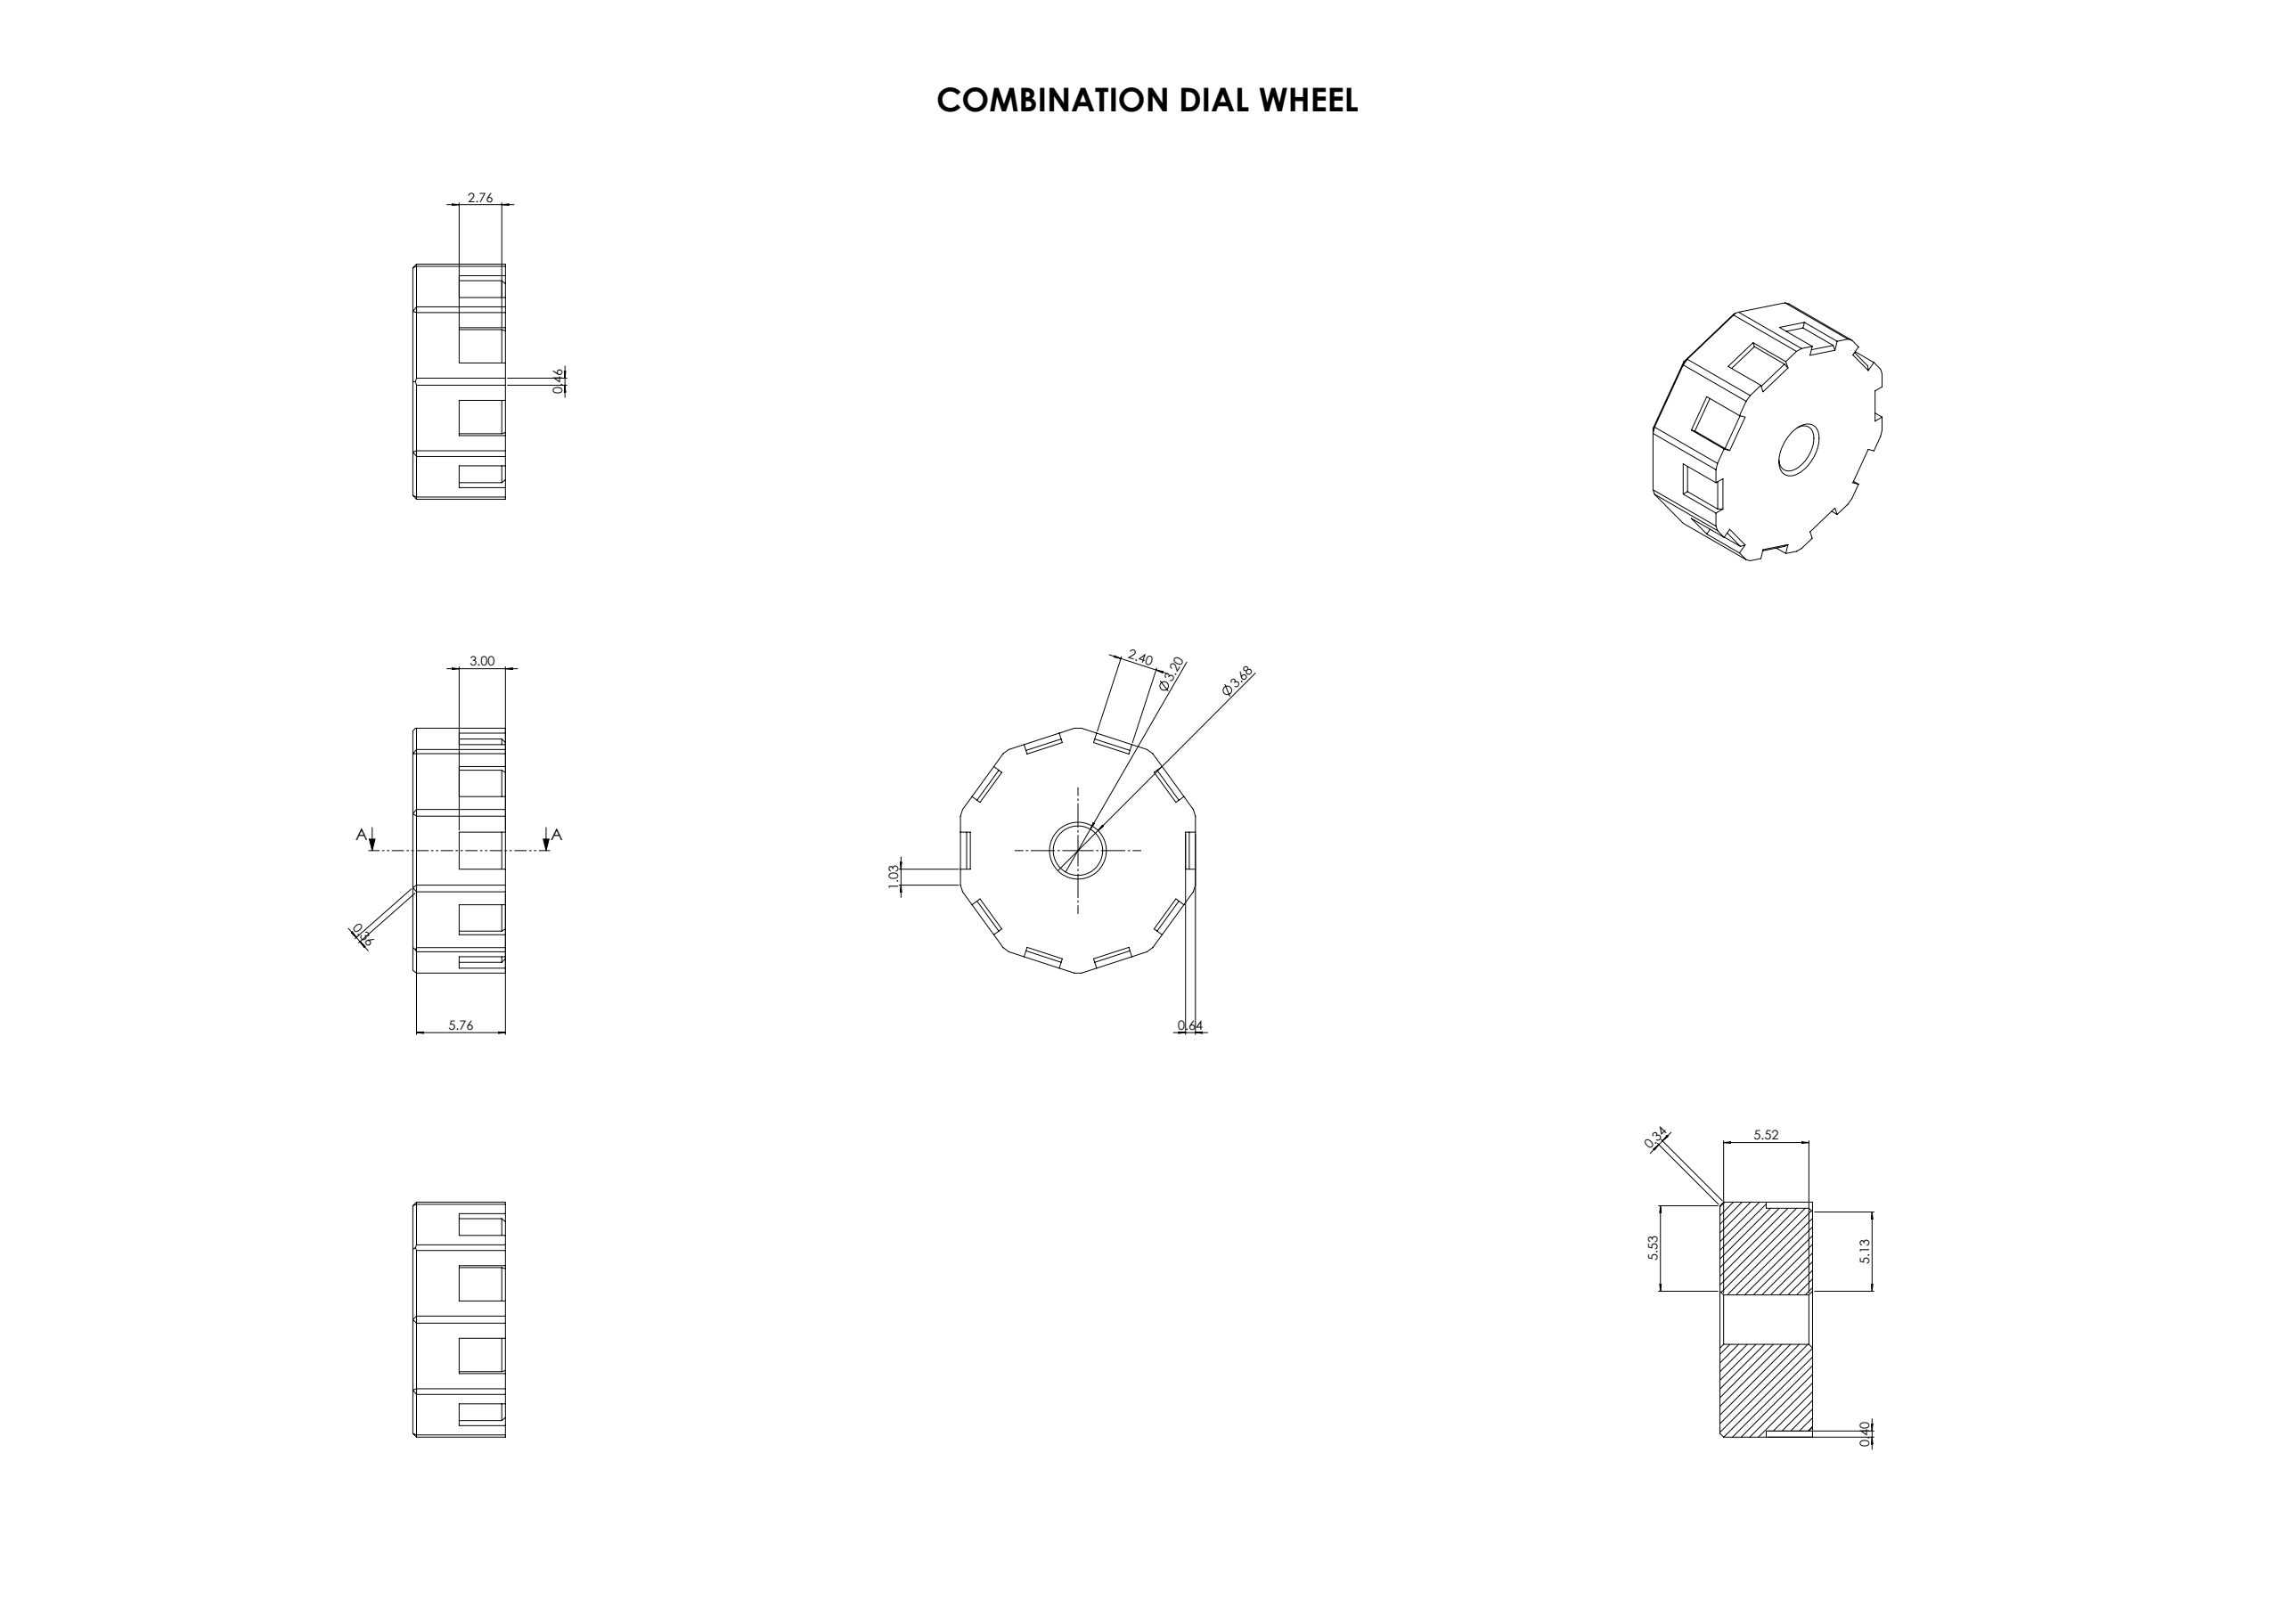
ISO-10303-21;
HEADER;
/* Generated by software containing ST-Developer
 * from STEP Tools, Inc. (www.steptools.com) 
 */

FILE_DESCRIPTION(
/* description */ (''),
/* implementation_level */ '2;1');

FILE_NAME(
/* name */ '10_Combination_Dial_Wheel.step',
/* time_stamp */ '2026-10-25T01:30:15-07:00',
/* author */ (''),
/* organization */ (''),
/* preprocessor_version */ 'ST-DEVELOPER v20.2',
/* originating_system */ 'Autodesk Translation Framework v15.15.0.0',
/* authorisation */ '');

FILE_SCHEMA (('AUTOMOTIVE_DESIGN { 1 0 10303 214 3 1 1 }'));
ENDSEC;

DATA;
#10=MECHANICAL_DESIGN_GEOMETRIC_PRESENTATION_REPRESENTATION('',(#576),#32309);
#548=SHAPE_REPRESENTATION_RELATIONSHIP('SRR','None',#32375,#562);
#562=ADVANCED_BREP_SHAPE_REPRESENTATION('',(#590),#32308);
#576=STYLED_ITEM('',(#32488),#590);
#590=MANIFOLD_SOLID_BREP('Body1',#13817);
#645=FACE_BOUND('',#2804,.T.);
#646=FACE_BOUND('',#2807,.T.);
#772=CYLINDRICAL_SURFACE('',#14893,1.6);
#1093=CIRCLE('',#14891,1.6);
#1094=CIRCLE('',#14892,1.84);
#1095=CIRCLE('',#14894,1.6);
#1096=CIRCLE('',#14897,1.84);
#1240=CONICAL_SURFACE('',#14890,1.72,0.785398163397448);
#1241=CONICAL_SURFACE('',#14896,1.72,0.785398163397448);
#1948=FACE_OUTER_BOUND('',#2801,.T.);
#1949=FACE_OUTER_BOUND('',#2802,.T.);
#1950=FACE_OUTER_BOUND('',#2803,.T.);
#1951=FACE_OUTER_BOUND('',#2805,.T.);
#1952=FACE_OUTER_BOUND('',#2806,.T.);
#1953=FACE_OUTER_BOUND('',#2808,.T.);
#1954=FACE_OUTER_BOUND('',#2809,.T.);
#1955=FACE_OUTER_BOUND('',#2810,.T.);
#1956=FACE_OUTER_BOUND('',#2811,.T.);
#1957=FACE_OUTER_BOUND('',#2812,.T.);
#1958=FACE_OUTER_BOUND('',#2813,.T.);
#1959=FACE_OUTER_BOUND('',#2814,.T.);
#1960=FACE_OUTER_BOUND('',#2815,.T.);
#1961=FACE_OUTER_BOUND('',#2816,.T.);
#1962=FACE_OUTER_BOUND('',#2817,.T.);
#1963=FACE_OUTER_BOUND('',#2818,.T.);
#1964=FACE_OUTER_BOUND('',#2819,.T.);
#1965=FACE_OUTER_BOUND('',#2820,.T.);
#1966=FACE_OUTER_BOUND('',#2821,.T.);
#1967=FACE_OUTER_BOUND('',#2822,.T.);
#1968=FACE_OUTER_BOUND('',#2823,.T.);
#1969=FACE_OUTER_BOUND('',#2824,.T.);
#1970=FACE_OUTER_BOUND('',#2825,.T.);
#1971=FACE_OUTER_BOUND('',#2826,.T.);
#1972=FACE_OUTER_BOUND('',#2827,.T.);
#1973=FACE_OUTER_BOUND('',#2828,.T.);
#1974=FACE_OUTER_BOUND('',#2829,.T.);
#1975=FACE_OUTER_BOUND('',#2830,.T.);
#1976=FACE_OUTER_BOUND('',#2831,.T.);
#1977=FACE_OUTER_BOUND('',#2832,.T.);
#1978=FACE_OUTER_BOUND('',#2833,.T.);
#1979=FACE_OUTER_BOUND('',#2834,.T.);
#1980=FACE_OUTER_BOUND('',#2835,.T.);
#1981=FACE_OUTER_BOUND('',#2836,.T.);
#1982=FACE_OUTER_BOUND('',#2837,.T.);
#1983=FACE_OUTER_BOUND('',#2838,.T.);
#1984=FACE_OUTER_BOUND('',#2839,.T.);
#1985=FACE_OUTER_BOUND('',#2840,.T.);
#1986=FACE_OUTER_BOUND('',#2841,.T.);
#1987=FACE_OUTER_BOUND('',#2842,.T.);
#1988=FACE_OUTER_BOUND('',#2843,.T.);
#1989=FACE_OUTER_BOUND('',#2844,.T.);
#1990=FACE_OUTER_BOUND('',#2845,.T.);
#1991=FACE_OUTER_BOUND('',#2846,.T.);
#1992=FACE_OUTER_BOUND('',#2847,.T.);
#1993=FACE_OUTER_BOUND('',#2848,.T.);
#1994=FACE_OUTER_BOUND('',#2849,.T.);
#1995=FACE_OUTER_BOUND('',#2850,.T.);
#1996=FACE_OUTER_BOUND('',#2851,.T.);
#1997=FACE_OUTER_BOUND('',#2852,.T.);
#1998=FACE_OUTER_BOUND('',#2853,.T.);
#1999=FACE_OUTER_BOUND('',#2854,.T.);
#2000=FACE_OUTER_BOUND('',#2855,.T.);
#2001=FACE_OUTER_BOUND('',#2856,.T.);
#2002=FACE_OUTER_BOUND('',#2857,.T.);
#2003=FACE_OUTER_BOUND('',#2858,.T.);
#2004=FACE_OUTER_BOUND('',#2859,.T.);
#2005=FACE_OUTER_BOUND('',#2860,.T.);
#2006=FACE_OUTER_BOUND('',#2861,.T.);
#2007=FACE_OUTER_BOUND('',#2862,.T.);
#2008=FACE_OUTER_BOUND('',#2863,.T.);
#2009=FACE_OUTER_BOUND('',#2864,.T.);
#2010=FACE_OUTER_BOUND('',#2865,.T.);
#2011=FACE_OUTER_BOUND('',#2866,.T.);
#2012=FACE_OUTER_BOUND('',#2867,.T.);
#2013=FACE_OUTER_BOUND('',#2868,.T.);
#2014=FACE_OUTER_BOUND('',#2869,.T.);
#2015=FACE_OUTER_BOUND('',#2870,.T.);
#2016=FACE_OUTER_BOUND('',#2871,.T.);
#2017=FACE_OUTER_BOUND('',#2872,.T.);
#2018=FACE_OUTER_BOUND('',#2873,.T.);
#2019=FACE_OUTER_BOUND('',#2874,.T.);
#2020=FACE_OUTER_BOUND('',#2875,.T.);
#2021=FACE_OUTER_BOUND('',#2876,.T.);
#2022=FACE_OUTER_BOUND('',#2877,.T.);
#2023=FACE_OUTER_BOUND('',#2878,.T.);
#2024=FACE_OUTER_BOUND('',#2879,.T.);
#2025=FACE_OUTER_BOUND('',#2880,.T.);
#2026=FACE_OUTER_BOUND('',#2881,.T.);
#2027=FACE_OUTER_BOUND('',#2882,.T.);
#2028=FACE_OUTER_BOUND('',#2883,.T.);
#2029=FACE_OUTER_BOUND('',#2884,.T.);
#2030=FACE_OUTER_BOUND('',#2885,.T.);
#2031=FACE_OUTER_BOUND('',#2886,.T.);
#2032=FACE_OUTER_BOUND('',#2887,.T.);
#2033=FACE_OUTER_BOUND('',#2888,.T.);
#2034=FACE_OUTER_BOUND('',#2889,.T.);
#2035=FACE_OUTER_BOUND('',#2890,.T.);
#2036=FACE_OUTER_BOUND('',#2891,.T.);
#2037=FACE_OUTER_BOUND('',#2892,.T.);
#2038=FACE_OUTER_BOUND('',#2893,.T.);
#2039=FACE_OUTER_BOUND('',#2894,.T.);
#2040=FACE_OUTER_BOUND('',#2895,.T.);
#2801=EDGE_LOOP('',(#12111,#12112,#12113,#12114));
#2802=EDGE_LOOP('',(#12115,#12116,#12117,#12118));
#2803=EDGE_LOOP('',(#12119,#12120,#12121,#12122,#12123,#12124,#12125,#12126,
#12127,#12128));
#2804=EDGE_LOOP('',(#12129));
#2805=EDGE_LOOP('',(#12130,#12131,#12132,#12133));
#2806=EDGE_LOOP('',(#12134,#12135,#12136,#12137,#12138,#12139,#12140,#12141,
#12142,#12143,#12144,#12145,#12146,#12147,#12148,#12149,#12150,#12151,#12152,
#12153,#12154,#12155,#12156,#12157,#12158,#12159,#12160,#12161,#12162,#12163,
#12164,#12165,#12166,#12167,#12168,#12169,#12170,#12171,#12172,#12173,#12174,
#12175,#12176,#12177,#12178,#12179,#12180,#12181,#12182,#12183,#12184,#12185,
#12186,#12187,#12188,#12189,#12190,#12191,#12192,#12193));
#2807=EDGE_LOOP('',(#12194));
#2808=EDGE_LOOP('',(#12195,#12196,#12197,#12198));
#2809=EDGE_LOOP('',(#12199,#12200,#12201,#12202));
#2810=EDGE_LOOP('',(#12203,#12204,#12205,#12206));
#2811=EDGE_LOOP('',(#12207,#12208,#12209,#12210));
#2812=EDGE_LOOP('',(#12211,#12212,#12213,#12214));
#2813=EDGE_LOOP('',(#12215,#12216,#12217,#12218));
#2814=EDGE_LOOP('',(#12219,#12220,#12221));
#2815=EDGE_LOOP('',(#12222,#12223,#12224,#12225,#12226));
#2816=EDGE_LOOP('',(#12227,#12228,#12229));
#2817=EDGE_LOOP('',(#12230,#12231,#12232,#12233));
#2818=EDGE_LOOP('',(#12234,#12235,#12236));
#2819=EDGE_LOOP('',(#12237,#12238,#12239,#12240));
#2820=EDGE_LOOP('',(#12241,#12242,#12243,#12244,#12245));
#2821=EDGE_LOOP('',(#12246,#12247,#12248,#12249));
#2822=EDGE_LOOP('',(#12250,#12251,#12252,#12253));
#2823=EDGE_LOOP('',(#12254,#12255,#12256,#12257));
#2824=EDGE_LOOP('',(#12258,#12259,#12260,#12261,#12262,#12263,#12264,#12265));
#2825=EDGE_LOOP('',(#12266,#12267,#12268,#12269,#12270,#12271,#12272,#12273));
#2826=EDGE_LOOP('',(#12274,#12275,#12276,#12277,#12278,#12279,#12280,#12281));
#2827=EDGE_LOOP('',(#12282,#12283,#12284,#12285,#12286));
#2828=EDGE_LOOP('',(#12287,#12288,#12289,#12290,#12291));
#2829=EDGE_LOOP('',(#12292,#12293,#12294,#12295));
#2830=EDGE_LOOP('',(#12296,#12297,#12298,#12299));
#2831=EDGE_LOOP('',(#12300,#12301,#12302,#12303));
#2832=EDGE_LOOP('',(#12304,#12305,#12306,#12307));
#2833=EDGE_LOOP('',(#12308,#12309,#12310,#12311));
#2834=EDGE_LOOP('',(#12312,#12313,#12314,#12315));
#2835=EDGE_LOOP('',(#12316,#12317,#12318,#12319));
#2836=EDGE_LOOP('',(#12320,#12321,#12322,#12323));
#2837=EDGE_LOOP('',(#12324,#12325,#12326,#12327));
#2838=EDGE_LOOP('',(#12328,#12329,#12330,#12331));
#2839=EDGE_LOOP('',(#12332,#12333,#12334,#12335));
#2840=EDGE_LOOP('',(#12336,#12337,#12338,#12339));
#2841=EDGE_LOOP('',(#12340,#12341,#12342));
#2842=EDGE_LOOP('',(#12343,#12344,#12345));
#2843=EDGE_LOOP('',(#12346,#12347,#12348,#12349));
#2844=EDGE_LOOP('',(#12350,#12351,#12352));
#2845=EDGE_LOOP('',(#12353,#12354,#12355,#12356));
#2846=EDGE_LOOP('',(#12357,#12358,#12359));
#2847=EDGE_LOOP('',(#12360,#12361,#12362,#12363));
#2848=EDGE_LOOP('',(#12364,#12365,#12366));
#2849=EDGE_LOOP('',(#12367,#12368,#12369,#12370,#12371));
#2850=EDGE_LOOP('',(#12372,#12373,#12374,#12375));
#2851=EDGE_LOOP('',(#12376,#12377,#12378,#12379));
#2852=EDGE_LOOP('',(#12380,#12381,#12382,#12383,#12384));
#2853=EDGE_LOOP('',(#12385,#12386,#12387,#12388));
#2854=EDGE_LOOP('',(#12389,#12390,#12391,#12392));
#2855=EDGE_LOOP('',(#12393,#12394,#12395,#12396));
#2856=EDGE_LOOP('',(#12397,#12398,#12399,#12400));
#2857=EDGE_LOOP('',(#12401,#12402,#12403,#12404,#12405,#12406,#12407,#12408));
#2858=EDGE_LOOP('',(#12409,#12410,#12411,#12412,#12413,#12414,#12415,#12416));
#2859=EDGE_LOOP('',(#12417,#12418,#12419,#12420,#12421,#12422,#12423,#12424));
#2860=EDGE_LOOP('',(#12425,#12426,#12427,#12428,#12429,#12430,#12431,#12432));
#2861=EDGE_LOOP('',(#12433,#12434,#12435,#12436,#12437,#12438,#12439,#12440));
#2862=EDGE_LOOP('',(#12441,#12442,#12443,#12444));
#2863=EDGE_LOOP('',(#12445,#12446,#12447,#12448));
#2864=EDGE_LOOP('',(#12449,#12450,#12451,#12452));
#2865=EDGE_LOOP('',(#12453,#12454,#12455,#12456,#12457));
#2866=EDGE_LOOP('',(#12458,#12459,#12460,#12461,#12462));
#2867=EDGE_LOOP('',(#12463,#12464,#12465,#12466,#12467,#12468,#12469,#12470));
#2868=EDGE_LOOP('',(#12471,#12472,#12473,#12474));
#2869=EDGE_LOOP('',(#12475,#12476,#12477,#12478,#12479));
#2870=EDGE_LOOP('',(#12480,#12481,#12482,#12483,#12484));
#2871=EDGE_LOOP('',(#12485,#12486,#12487,#12488));
#2872=EDGE_LOOP('',(#12489,#12490,#12491,#12492,#12493));
#2873=EDGE_LOOP('',(#12494,#12495,#12496,#12497,#12498));
#2874=EDGE_LOOP('',(#12499,#12500,#12501,#12502));
#2875=EDGE_LOOP('',(#12503,#12504,#12505,#12506,#12507));
#2876=EDGE_LOOP('',(#12508,#12509,#12510,#12511,#12512));
#2877=EDGE_LOOP('',(#12513,#12514,#12515,#12516));
#2878=EDGE_LOOP('',(#12517,#12518,#12519,#12520,#12521));
#2879=EDGE_LOOP('',(#12522,#12523,#12524,#12525,#12526));
#2880=EDGE_LOOP('',(#12527,#12528,#12529,#12530));
#2881=EDGE_LOOP('',(#12531,#12532,#12533,#12534,#12535));
#2882=EDGE_LOOP('',(#12536,#12537,#12538,#12539,#12540));
#2883=EDGE_LOOP('',(#12541,#12542,#12543,#12544));
#2884=EDGE_LOOP('',(#12545,#12546,#12547,#12548,#12549));
#2885=EDGE_LOOP('',(#12550,#12551,#12552,#12553,#12554));
#2886=EDGE_LOOP('',(#12555,#12556,#12557,#12558));
#2887=EDGE_LOOP('',(#12559,#12560,#12561,#12562,#12563));
#2888=EDGE_LOOP('',(#12564,#12565,#12566,#12567,#12568));
#2889=EDGE_LOOP('',(#12569,#12570,#12571,#12572));
#2890=EDGE_LOOP('',(#12573,#12574,#12575,#12576,#12577));
#2891=EDGE_LOOP('',(#12578,#12579,#12580,#12581,#12582));
#2892=EDGE_LOOP('',(#12583,#12584,#12585,#12586,#12587));
#2893=EDGE_LOOP('',(#12588,#12589,#12590,#12591,#12592));
#2894=EDGE_LOOP('',(#12593,#12594,#12595,#12596));
#2895=EDGE_LOOP('',(#12597,#12598,#12599,#12600,#12601,#12602,#12603,#12604));
#3964=LINE('',#31769,#5275);
#3965=LINE('',#31774,#5276);
#3966=LINE('',#31778,#5277);
#3967=LINE('',#31780,#5278);
#3968=LINE('',#31782,#5279);
#3969=LINE('',#31784,#5280);
#3970=LINE('',#31786,#5281);
#3971=LINE('',#31788,#5282);
#3972=LINE('',#31790,#5283);
#3973=LINE('',#31792,#5284);
#3974=LINE('',#31794,#5285);
#3975=LINE('',#31795,#5286);
#3976=LINE('',#31799,#5287);
#3977=LINE('',#31803,#5288);
#3978=LINE('',#31805,#5289);
#3979=LINE('',#31807,#5290);
#3980=LINE('',#31809,#5291);
#3981=LINE('',#31811,#5292);
#3982=LINE('',#31813,#5293);
#3983=LINE('',#31815,#5294);
#3984=LINE('',#31817,#5295);
#3985=LINE('',#31819,#5296);
#3986=LINE('',#31821,#5297);
#3987=LINE('',#31823,#5298);
#3988=LINE('',#31825,#5299);
#3989=LINE('',#31827,#5300);
#3990=LINE('',#31829,#5301);
#3991=LINE('',#31831,#5302);
#3992=LINE('',#31833,#5303);
#3993=LINE('',#31835,#5304);
#3994=LINE('',#31837,#5305);
#3995=LINE('',#31839,#5306);
#3996=LINE('',#31841,#5307);
#3997=LINE('',#31843,#5308);
#3998=LINE('',#31845,#5309);
#3999=LINE('',#31847,#5310);
#4000=LINE('',#31849,#5311);
#4001=LINE('',#31851,#5312);
#4002=LINE('',#31853,#5313);
#4003=LINE('',#31855,#5314);
#4004=LINE('',#31857,#5315);
#4005=LINE('',#31859,#5316);
#4006=LINE('',#31861,#5317);
#4007=LINE('',#31863,#5318);
#4008=LINE('',#31865,#5319);
#4009=LINE('',#31867,#5320);
#4010=LINE('',#31869,#5321);
#4011=LINE('',#31871,#5322);
#4012=LINE('',#31873,#5323);
#4013=LINE('',#31875,#5324);
#4014=LINE('',#31877,#5325);
#4015=LINE('',#31879,#5326);
#4016=LINE('',#31881,#5327);
#4017=LINE('',#31883,#5328);
#4018=LINE('',#31885,#5329);
#4019=LINE('',#31887,#5330);
#4020=LINE('',#31889,#5331);
#4021=LINE('',#31891,#5332);
#4022=LINE('',#31893,#5333);
#4023=LINE('',#31895,#5334);
#4024=LINE('',#31897,#5335);
#4025=LINE('',#31899,#5336);
#4026=LINE('',#31901,#5337);
#4027=LINE('',#31903,#5338);
#4028=LINE('',#31905,#5339);
#4029=LINE('',#31907,#5340);
#4030=LINE('',#31909,#5341);
#4031=LINE('',#31911,#5342);
#4032=LINE('',#31913,#5343);
#4033=LINE('',#31915,#5344);
#4034=LINE('',#31917,#5345);
#4035=LINE('',#31919,#5346);
#4036=LINE('',#31920,#5347);
#4037=LINE('',#31923,#5348);
#4038=LINE('',#31925,#5349);
#4039=LINE('',#31926,#5350);
#4040=LINE('',#31929,#5351);
#4041=LINE('',#31931,#5352);
#4042=LINE('',#31932,#5353);
#4043=LINE('',#31935,#5354);
#4044=LINE('',#31937,#5355);
#4045=LINE('',#31938,#5356);
#4046=LINE('',#31941,#5357);
#4047=LINE('',#31943,#5358);
#4048=LINE('',#31944,#5359);
#4049=LINE('',#31947,#5360);
#4050=LINE('',#31949,#5361);
#4051=LINE('',#31950,#5362);
#4052=LINE('',#31953,#5363);
#4053=LINE('',#31955,#5364);
#4054=LINE('',#31956,#5365);
#4055=LINE('',#31960,#5366);
#4056=LINE('',#31961,#5367);
#4057=LINE('',#31962,#5368);
#4058=LINE('',#31965,#5369);
#4059=LINE('',#31967,#5370);
#4060=LINE('',#31968,#5371);
#4061=LINE('',#31972,#5372);
#4062=LINE('',#31973,#5373);
#4063=LINE('',#31974,#5374);
#4064=LINE('',#31976,#5375);
#4065=LINE('',#31980,#5376);
#4066=LINE('',#31981,#5377);
#4067=LINE('',#31982,#5378);
#4068=LINE('',#31984,#5379);
#4069=LINE('',#31988,#5380);
#4070=LINE('',#31989,#5381);
#4071=LINE('',#31990,#5382);
#4072=LINE('',#31992,#5383);
#4073=LINE('',#31993,#5384);
#4074=LINE('',#31995,#5385);
#4075=LINE('',#31996,#5386);
#4076=LINE('',#31998,#5387);
#4077=LINE('',#31999,#5388);
#4078=LINE('',#32002,#5389);
#4079=LINE('',#32004,#5390);
#4080=LINE('',#32005,#5391);
#4081=LINE('',#32008,#5392);
#4082=LINE('',#32010,#5393);
#4083=LINE('',#32011,#5394);
#4084=LINE('',#32013,#5395);
#4085=LINE('',#32015,#5396);
#4086=LINE('',#32017,#5397);
#4087=LINE('',#32018,#5398);
#4088=LINE('',#32021,#5399);
#4089=LINE('',#32022,#5400);
#4090=LINE('',#32025,#5401);
#4091=LINE('',#32026,#5402);
#4092=LINE('',#32029,#5403);
#4093=LINE('',#32031,#5404);
#4094=LINE('',#32032,#5405);
#4095=LINE('',#32035,#5406);
#4096=LINE('',#32037,#5407);
#4097=LINE('',#32038,#5408);
#4098=LINE('',#32041,#5409);
#4099=LINE('',#32043,#5410);
#4100=LINE('',#32044,#5411);
#4101=LINE('',#32047,#5412);
#4102=LINE('',#32049,#5413);
#4103=LINE('',#32050,#5414);
#4104=LINE('',#32053,#5415);
#4105=LINE('',#32055,#5416);
#4106=LINE('',#32056,#5417);
#4107=LINE('',#32059,#5418);
#4108=LINE('',#32061,#5419);
#4109=LINE('',#32062,#5420);
#4110=LINE('',#32065,#5421);
#4111=LINE('',#32067,#5422);
#4112=LINE('',#32068,#5423);
#4113=LINE('',#32071,#5424);
#4114=LINE('',#32073,#5425);
#4115=LINE('',#32074,#5426);
#4116=LINE('',#32077,#5427);
#4117=LINE('',#32079,#5428);
#4118=LINE('',#32080,#5429);
#4119=LINE('',#32083,#5430);
#4120=LINE('',#32085,#5431);
#4121=LINE('',#32086,#5432);
#4122=LINE('',#32089,#5433);
#4123=LINE('',#32091,#5434);
#4124=LINE('',#32092,#5435);
#4125=LINE('',#32095,#5436);
#4126=LINE('',#32097,#5437);
#4127=LINE('',#32098,#5438);
#4128=LINE('',#32101,#5439);
#4129=LINE('',#32102,#5440);
#4130=LINE('',#32106,#5441);
#4131=LINE('',#32107,#5442);
#4132=LINE('',#32108,#5443);
#4133=LINE('',#32110,#5444);
#4134=LINE('',#32114,#5445);
#4135=LINE('',#32115,#5446);
#4136=LINE('',#32116,#5447);
#4137=LINE('',#32118,#5448);
#4138=LINE('',#32122,#5449);
#4139=LINE('',#32123,#5450);
#4140=LINE('',#32124,#5451);
#4141=LINE('',#32126,#5452);
#4142=LINE('',#32129,#5453);
#4143=LINE('',#32131,#5454);
#4144=LINE('',#32132,#5455);
#4145=LINE('',#32135,#5456);
#4146=LINE('',#32136,#5457);
#4147=LINE('',#32138,#5458);
#4148=LINE('',#32139,#5459);
#4149=LINE('',#32141,#5460);
#4150=LINE('',#32143,#5461);
#4151=LINE('',#32144,#5462);
#4152=LINE('',#32146,#5463);
#4153=LINE('',#32147,#5464);
#4154=LINE('',#32149,#5465);
#4155=LINE('',#32150,#5466);
#4156=LINE('',#32152,#5467);
#4157=LINE('',#32153,#5468);
#4158=LINE('',#32155,#5469);
#4159=LINE('',#32156,#5470);
#4160=LINE('',#32159,#5471);
#4161=LINE('',#32161,#5472);
#4162=LINE('',#32162,#5473);
#4163=LINE('',#32165,#5474);
#4164=LINE('',#32167,#5475);
#4165=LINE('',#32168,#5476);
#4166=LINE('',#32171,#5477);
#4167=LINE('',#32173,#5478);
#4168=LINE('',#32174,#5479);
#4169=LINE('',#32177,#5480);
#4170=LINE('',#32179,#5481);
#4171=LINE('',#32180,#5482);
#4172=LINE('',#32183,#5483);
#4173=LINE('',#32185,#5484);
#4174=LINE('',#32186,#5485);
#4175=LINE('',#32189,#5486);
#4176=LINE('',#32191,#5487);
#4177=LINE('',#32192,#5488);
#4178=LINE('',#32195,#5489);
#4179=LINE('',#32197,#5490);
#4180=LINE('',#32198,#5491);
#4181=LINE('',#32202,#5492);
#4182=LINE('',#32203,#5493);
#4183=LINE('',#32204,#5494);
#4184=LINE('',#32206,#5495);
#4185=LINE('',#32208,#5496);
#4186=LINE('',#32211,#5497);
#4187=LINE('',#32212,#5498);
#4188=LINE('',#32216,#5499);
#4189=LINE('',#32217,#5500);
#4190=LINE('',#32221,#5501);
#4191=LINE('',#32222,#5502);
#4192=LINE('',#32226,#5503);
#4193=LINE('',#32227,#5504);
#4194=LINE('',#32231,#5505);
#4195=LINE('',#32232,#5506);
#4196=LINE('',#32236,#5507);
#4197=LINE('',#32237,#5508);
#4198=LINE('',#32241,#5509);
#4199=LINE('',#32242,#5510);
#4200=LINE('',#32246,#5511);
#4201=LINE('',#32247,#5512);
#4202=LINE('',#32252,#5513);
#4203=LINE('',#32253,#5514);
#4204=LINE('',#32256,#5515);
#4205=LINE('',#32257,#5516);
#4206=LINE('',#32259,#5517);
#5275=VECTOR('',#17910,1.72);
#5276=VECTOR('',#17917,1.6);
#5277=VECTOR('',#17920,10.);
#5278=VECTOR('',#17921,10.);
#5279=VECTOR('',#17922,10.);
#5280=VECTOR('',#17923,10.);
#5281=VECTOR('',#17924,10.);
#5282=VECTOR('',#17925,10.);
#5283=VECTOR('',#17926,10.);
#5284=VECTOR('',#17927,10.);
#5285=VECTOR('',#17928,10.);
#5286=VECTOR('',#17929,10.);
#5287=VECTOR('',#17934,1.72);
#5288=VECTOR('',#17937,10.);
#5289=VECTOR('',#17938,10.);
#5290=VECTOR('',#17939,10.);
#5291=VECTOR('',#17940,10.);
#5292=VECTOR('',#17941,10.);
#5293=VECTOR('',#17942,10.);
#5294=VECTOR('',#17943,10.);
#5295=VECTOR('',#17944,10.);
#5296=VECTOR('',#17945,10.);
#5297=VECTOR('',#17946,10.);
#5298=VECTOR('',#17947,10.);
#5299=VECTOR('',#17948,10.);
#5300=VECTOR('',#17949,10.);
#5301=VECTOR('',#17950,10.);
#5302=VECTOR('',#17951,10.);
#5303=VECTOR('',#17952,10.);
#5304=VECTOR('',#17953,10.);
#5305=VECTOR('',#17954,10.);
#5306=VECTOR('',#17955,10.);
#5307=VECTOR('',#17956,10.);
#5308=VECTOR('',#17957,10.);
#5309=VECTOR('',#17958,10.);
#5310=VECTOR('',#17959,10.);
#5311=VECTOR('',#17960,10.);
#5312=VECTOR('',#17961,10.);
#5313=VECTOR('',#17962,10.);
#5314=VECTOR('',#17963,10.);
#5315=VECTOR('',#17964,10.);
#5316=VECTOR('',#17965,10.);
#5317=VECTOR('',#17966,10.);
#5318=VECTOR('',#17967,10.);
#5319=VECTOR('',#17968,10.);
#5320=VECTOR('',#17969,10.);
#5321=VECTOR('',#17970,10.);
#5322=VECTOR('',#17971,10.);
#5323=VECTOR('',#17972,10.);
#5324=VECTOR('',#17973,10.);
#5325=VECTOR('',#17974,10.);
#5326=VECTOR('',#17975,10.);
#5327=VECTOR('',#17976,10.);
#5328=VECTOR('',#17977,10.);
#5329=VECTOR('',#17978,10.);
#5330=VECTOR('',#17979,10.);
#5331=VECTOR('',#17980,10.);
#5332=VECTOR('',#17981,10.);
#5333=VECTOR('',#17982,10.);
#5334=VECTOR('',#17983,10.);
#5335=VECTOR('',#17984,10.);
#5336=VECTOR('',#17985,10.);
#5337=VECTOR('',#17986,10.);
#5338=VECTOR('',#17987,10.);
#5339=VECTOR('',#17988,10.);
#5340=VECTOR('',#17989,10.);
#5341=VECTOR('',#17990,10.);
#5342=VECTOR('',#17991,10.);
#5343=VECTOR('',#17992,10.);
#5344=VECTOR('',#17993,10.);
#5345=VECTOR('',#17994,10.);
#5346=VECTOR('',#17995,10.);
#5347=VECTOR('',#17996,10.);
#5348=VECTOR('',#17999,10.);
#5349=VECTOR('',#18000,10.);
#5350=VECTOR('',#18001,10.);
#5351=VECTOR('',#18004,10.);
#5352=VECTOR('',#18005,10.);
#5353=VECTOR('',#18006,10.);
#5354=VECTOR('',#18009,10.);
#5355=VECTOR('',#18010,10.);
#5356=VECTOR('',#18011,10.);
#5357=VECTOR('',#18014,10.);
#5358=VECTOR('',#18015,10.);
#5359=VECTOR('',#18016,10.);
#5360=VECTOR('',#18019,10.);
#5361=VECTOR('',#18020,10.);
#5362=VECTOR('',#18021,10.);
#5363=VECTOR('',#18024,10.);
#5364=VECTOR('',#18025,10.);
#5365=VECTOR('',#18026,10.);
#5366=VECTOR('',#18029,10.);
#5367=VECTOR('',#18030,10.);
#5368=VECTOR('',#18031,10.);
#5369=VECTOR('',#18034,10.);
#5370=VECTOR('',#18035,10.);
#5371=VECTOR('',#18036,10.);
#5372=VECTOR('',#18039,10.);
#5373=VECTOR('',#18040,10.);
#5374=VECTOR('',#18041,10.);
#5375=VECTOR('',#18044,10.);
#5376=VECTOR('',#18047,10.);
#5377=VECTOR('',#18048,10.);
#5378=VECTOR('',#18049,10.);
#5379=VECTOR('',#18052,10.);
#5380=VECTOR('',#18055,10.);
#5381=VECTOR('',#18056,10.);
#5382=VECTOR('',#18057,10.);
#5383=VECTOR('',#18060,10.);
#5384=VECTOR('',#18061,10.);
#5385=VECTOR('',#18064,10.);
#5386=VECTOR('',#18065,10.);
#5387=VECTOR('',#18068,10.);
#5388=VECTOR('',#18069,10.);
#5389=VECTOR('',#18072,10.);
#5390=VECTOR('',#18073,10.);
#5391=VECTOR('',#18074,10.);
#5392=VECTOR('',#18077,10.);
#5393=VECTOR('',#18078,10.);
#5394=VECTOR('',#18079,10.);
#5395=VECTOR('',#18082,10.);
#5396=VECTOR('',#18083,10.);
#5397=VECTOR('',#18084,10.);
#5398=VECTOR('',#18085,10.);
#5399=VECTOR('',#18088,10.);
#5400=VECTOR('',#18089,10.);
#5401=VECTOR('',#18092,10.);
#5402=VECTOR('',#18093,10.);
#5403=VECTOR('',#18096,10.);
#5404=VECTOR('',#18097,10.);
#5405=VECTOR('',#18098,10.);
#5406=VECTOR('',#18101,10.);
#5407=VECTOR('',#18102,10.);
#5408=VECTOR('',#18103,10.);
#5409=VECTOR('',#18106,10.);
#5410=VECTOR('',#18107,10.);
#5411=VECTOR('',#18108,10.);
#5412=VECTOR('',#18111,10.);
#5413=VECTOR('',#18112,10.);
#5414=VECTOR('',#18113,10.);
#5415=VECTOR('',#18116,10.);
#5416=VECTOR('',#18117,10.);
#5417=VECTOR('',#18118,10.);
#5418=VECTOR('',#18121,10.);
#5419=VECTOR('',#18122,10.);
#5420=VECTOR('',#18123,10.);
#5421=VECTOR('',#18126,10.);
#5422=VECTOR('',#18127,10.);
#5423=VECTOR('',#18128,10.);
#5424=VECTOR('',#18131,10.);
#5425=VECTOR('',#18132,10.);
#5426=VECTOR('',#18133,10.);
#5427=VECTOR('',#18136,10.);
#5428=VECTOR('',#18137,10.);
#5429=VECTOR('',#18138,10.);
#5430=VECTOR('',#18141,10.);
#5431=VECTOR('',#18142,10.);
#5432=VECTOR('',#18143,10.);
#5433=VECTOR('',#18146,10.);
#5434=VECTOR('',#18147,10.);
#5435=VECTOR('',#18148,10.);
#5436=VECTOR('',#18151,10.);
#5437=VECTOR('',#18152,10.);
#5438=VECTOR('',#18153,10.);
#5439=VECTOR('',#18156,10.);
#5440=VECTOR('',#18157,10.);
#5441=VECTOR('',#18160,10.);
#5442=VECTOR('',#18161,10.);
#5443=VECTOR('',#18162,10.);
#5444=VECTOR('',#18165,10.);
#5445=VECTOR('',#18168,10.);
#5446=VECTOR('',#18169,10.);
#5447=VECTOR('',#18170,10.);
#5448=VECTOR('',#18173,10.);
#5449=VECTOR('',#18176,10.);
#5450=VECTOR('',#18177,10.);
#5451=VECTOR('',#18178,10.);
#5452=VECTOR('',#18181,10.);
#5453=VECTOR('',#18184,10.);
#5454=VECTOR('',#18185,10.);
#5455=VECTOR('',#18186,10.);
#5456=VECTOR('',#18189,10.);
#5457=VECTOR('',#18190,10.);
#5458=VECTOR('',#18193,10.);
#5459=VECTOR('',#18194,10.);
#5460=VECTOR('',#18197,10.);
#5461=VECTOR('',#18200,10.);
#5462=VECTOR('',#18201,10.);
#5463=VECTOR('',#18204,10.);
#5464=VECTOR('',#18205,10.);
#5465=VECTOR('',#18208,10.);
#5466=VECTOR('',#18209,10.);
#5467=VECTOR('',#18212,10.);
#5468=VECTOR('',#18213,10.);
#5469=VECTOR('',#18216,10.);
#5470=VECTOR('',#18217,10.);
#5471=VECTOR('',#18220,10.);
#5472=VECTOR('',#18221,10.);
#5473=VECTOR('',#18222,10.);
#5474=VECTOR('',#18225,10.);
#5475=VECTOR('',#18226,10.);
#5476=VECTOR('',#18227,10.);
#5477=VECTOR('',#18230,10.);
#5478=VECTOR('',#18231,10.);
#5479=VECTOR('',#18232,10.);
#5480=VECTOR('',#18235,10.);
#5481=VECTOR('',#18236,10.);
#5482=VECTOR('',#18237,10.);
#5483=VECTOR('',#18240,10.);
#5484=VECTOR('',#18241,10.);
#5485=VECTOR('',#18242,10.);
#5486=VECTOR('',#18245,10.);
#5487=VECTOR('',#18246,10.);
#5488=VECTOR('',#18247,10.);
#5489=VECTOR('',#18250,10.);
#5490=VECTOR('',#18251,10.);
#5491=VECTOR('',#18252,10.);
#5492=VECTOR('',#18255,10.);
#5493=VECTOR('',#18256,10.);
#5494=VECTOR('',#18257,10.);
#5495=VECTOR('',#18260,10.);
#5496=VECTOR('',#18263,10.);
#5497=VECTOR('',#18268,10.);
#5498=VECTOR('',#18269,10.);
#5499=VECTOR('',#18276,10.);
#5500=VECTOR('',#18277,10.);
#5501=VECTOR('',#18284,10.);
#5502=VECTOR('',#18285,10.);
#5503=VECTOR('',#18292,10.);
#5504=VECTOR('',#18293,10.);
#5505=VECTOR('',#18300,10.);
#5506=VECTOR('',#18301,10.);
#5507=VECTOR('',#18308,10.);
#5508=VECTOR('',#18309,10.);
#5509=VECTOR('',#18316,10.);
#5510=VECTOR('',#18317,10.);
#5511=VECTOR('',#18324,10.);
#5512=VECTOR('',#18325,10.);
#5513=VECTOR('',#18332,10.);
#5514=VECTOR('',#18333,10.);
#5515=VECTOR('',#18336,10.);
#5516=VECTOR('',#18337,10.);
#5517=VECTOR('',#18340,10.);
#6560=VERTEX_POINT('',#31766);
#6561=VERTEX_POINT('',#31768);
#6562=VERTEX_POINT('',#31772);
#6563=VERTEX_POINT('',#31776);
#6564=VERTEX_POINT('',#31777);
#6565=VERTEX_POINT('',#31779);
#6566=VERTEX_POINT('',#31781);
#6567=VERTEX_POINT('',#31783);
#6568=VERTEX_POINT('',#31785);
#6569=VERTEX_POINT('',#31787);
#6570=VERTEX_POINT('',#31789);
#6571=VERTEX_POINT('',#31791);
#6572=VERTEX_POINT('',#31793);
#6573=VERTEX_POINT('',#31797);
#6574=VERTEX_POINT('',#31801);
#6575=VERTEX_POINT('',#31802);
#6576=VERTEX_POINT('',#31804);
#6577=VERTEX_POINT('',#31806);
#6578=VERTEX_POINT('',#31808);
#6579=VERTEX_POINT('',#31810);
#6580=VERTEX_POINT('',#31812);
#6581=VERTEX_POINT('',#31814);
#6582=VERTEX_POINT('',#31816);
#6583=VERTEX_POINT('',#31818);
#6584=VERTEX_POINT('',#31820);
#6585=VERTEX_POINT('',#31822);
#6586=VERTEX_POINT('',#31824);
#6587=VERTEX_POINT('',#31826);
#6588=VERTEX_POINT('',#31828);
#6589=VERTEX_POINT('',#31830);
#6590=VERTEX_POINT('',#31832);
#6591=VERTEX_POINT('',#31834);
#6592=VERTEX_POINT('',#31836);
#6593=VERTEX_POINT('',#31838);
#6594=VERTEX_POINT('',#31840);
#6595=VERTEX_POINT('',#31842);
#6596=VERTEX_POINT('',#31844);
#6597=VERTEX_POINT('',#31846);
#6598=VERTEX_POINT('',#31848);
#6599=VERTEX_POINT('',#31850);
#6600=VERTEX_POINT('',#31852);
#6601=VERTEX_POINT('',#31854);
#6602=VERTEX_POINT('',#31856);
#6603=VERTEX_POINT('',#31858);
#6604=VERTEX_POINT('',#31860);
#6605=VERTEX_POINT('',#31862);
#6606=VERTEX_POINT('',#31864);
#6607=VERTEX_POINT('',#31866);
#6608=VERTEX_POINT('',#31868);
#6609=VERTEX_POINT('',#31870);
#6610=VERTEX_POINT('',#31872);
#6611=VERTEX_POINT('',#31874);
#6612=VERTEX_POINT('',#31876);
#6613=VERTEX_POINT('',#31878);
#6614=VERTEX_POINT('',#31880);
#6615=VERTEX_POINT('',#31882);
#6616=VERTEX_POINT('',#31884);
#6617=VERTEX_POINT('',#31886);
#6618=VERTEX_POINT('',#31888);
#6619=VERTEX_POINT('',#31890);
#6620=VERTEX_POINT('',#31892);
#6621=VERTEX_POINT('',#31894);
#6622=VERTEX_POINT('',#31896);
#6623=VERTEX_POINT('',#31898);
#6624=VERTEX_POINT('',#31900);
#6625=VERTEX_POINT('',#31902);
#6626=VERTEX_POINT('',#31904);
#6627=VERTEX_POINT('',#31906);
#6628=VERTEX_POINT('',#31908);
#6629=VERTEX_POINT('',#31910);
#6630=VERTEX_POINT('',#31912);
#6631=VERTEX_POINT('',#31914);
#6632=VERTEX_POINT('',#31916);
#6633=VERTEX_POINT('',#31918);
#6634=VERTEX_POINT('',#31922);
#6635=VERTEX_POINT('',#31924);
#6636=VERTEX_POINT('',#31928);
#6637=VERTEX_POINT('',#31930);
#6638=VERTEX_POINT('',#31934);
#6639=VERTEX_POINT('',#31936);
#6640=VERTEX_POINT('',#31940);
#6641=VERTEX_POINT('',#31942);
#6642=VERTEX_POINT('',#31946);
#6643=VERTEX_POINT('',#31948);
#6644=VERTEX_POINT('',#31952);
#6645=VERTEX_POINT('',#31954);
#6646=VERTEX_POINT('',#31958);
#6647=VERTEX_POINT('',#31959);
#6648=VERTEX_POINT('',#31964);
#6649=VERTEX_POINT('',#31966);
#6650=VERTEX_POINT('',#31970);
#6651=VERTEX_POINT('',#31971);
#6652=VERTEX_POINT('',#31978);
#6653=VERTEX_POINT('',#31979);
#6654=VERTEX_POINT('',#31986);
#6655=VERTEX_POINT('',#31987);
#6656=VERTEX_POINT('',#32001);
#6657=VERTEX_POINT('',#32003);
#6658=VERTEX_POINT('',#32007);
#6659=VERTEX_POINT('',#32009);
#6660=VERTEX_POINT('',#32014);
#6661=VERTEX_POINT('',#32016);
#6662=VERTEX_POINT('',#32020);
#6663=VERTEX_POINT('',#32024);
#6664=VERTEX_POINT('',#32028);
#6665=VERTEX_POINT('',#32030);
#6666=VERTEX_POINT('',#32034);
#6667=VERTEX_POINT('',#32036);
#6668=VERTEX_POINT('',#32040);
#6669=VERTEX_POINT('',#32042);
#6670=VERTEX_POINT('',#32046);
#6671=VERTEX_POINT('',#32048);
#6672=VERTEX_POINT('',#32052);
#6673=VERTEX_POINT('',#32054);
#6674=VERTEX_POINT('',#32058);
#6675=VERTEX_POINT('',#32060);
#6676=VERTEX_POINT('',#32064);
#6677=VERTEX_POINT('',#32066);
#6678=VERTEX_POINT('',#32070);
#6679=VERTEX_POINT('',#32072);
#6680=VERTEX_POINT('',#32076);
#6681=VERTEX_POINT('',#32078);
#6682=VERTEX_POINT('',#32082);
#6683=VERTEX_POINT('',#32084);
#6684=VERTEX_POINT('',#32088);
#6685=VERTEX_POINT('',#32090);
#6686=VERTEX_POINT('',#32094);
#6687=VERTEX_POINT('',#32096);
#6688=VERTEX_POINT('',#32100);
#6689=VERTEX_POINT('',#32104);
#6690=VERTEX_POINT('',#32105);
#6691=VERTEX_POINT('',#32112);
#6692=VERTEX_POINT('',#32113);
#6693=VERTEX_POINT('',#32120);
#6694=VERTEX_POINT('',#32121);
#6695=VERTEX_POINT('',#32128);
#6696=VERTEX_POINT('',#32130);
#6697=VERTEX_POINT('',#32134);
#6698=VERTEX_POINT('',#32158);
#6699=VERTEX_POINT('',#32160);
#6700=VERTEX_POINT('',#32164);
#6701=VERTEX_POINT('',#32166);
#6702=VERTEX_POINT('',#32170);
#6703=VERTEX_POINT('',#32172);
#6704=VERTEX_POINT('',#32176);
#6705=VERTEX_POINT('',#32178);
#6706=VERTEX_POINT('',#32182);
#6707=VERTEX_POINT('',#32184);
#6708=VERTEX_POINT('',#32188);
#6709=VERTEX_POINT('',#32190);
#6710=VERTEX_POINT('',#32194);
#6711=VERTEX_POINT('',#32196);
#6712=VERTEX_POINT('',#32200);
#6713=VERTEX_POINT('',#32201);
#6714=VERTEX_POINT('',#32251);
#6715=VERTEX_POINT('',#32255);
#8432=EDGE_CURVE('',#6560,#6560,#1093,.T.);
#8433=EDGE_CURVE('',#6560,#6561,#3964,.T.);
#8434=EDGE_CURVE('',#6561,#6561,#1094,.T.);
#8435=EDGE_CURVE('',#6562,#6562,#1095,.T.);
#8436=EDGE_CURVE('',#6562,#6560,#3965,.T.);
#8437=EDGE_CURVE('',#6563,#6564,#3966,.T.);
#8438=EDGE_CURVE('',#6565,#6563,#3967,.T.);
#8439=EDGE_CURVE('',#6566,#6565,#3968,.T.);
#8440=EDGE_CURVE('',#6567,#6566,#3969,.T.);
#8441=EDGE_CURVE('',#6568,#6567,#3970,.T.);
#8442=EDGE_CURVE('',#6569,#6568,#3971,.T.);
#8443=EDGE_CURVE('',#6570,#6569,#3972,.T.);
#8444=EDGE_CURVE('',#6571,#6570,#3973,.T.);
#8445=EDGE_CURVE('',#6572,#6571,#3974,.T.);
#8446=EDGE_CURVE('',#6564,#6572,#3975,.T.);
#8447=EDGE_CURVE('',#6573,#6573,#1096,.T.);
#8448=EDGE_CURVE('',#6573,#6562,#3976,.T.);
#8449=EDGE_CURVE('',#6574,#6575,#3977,.T.);
#8450=EDGE_CURVE('',#6575,#6576,#3978,.T.);
#8451=EDGE_CURVE('',#6577,#6576,#3979,.T.);
#8452=EDGE_CURVE('',#6577,#6578,#3980,.T.);
#8453=EDGE_CURVE('',#6578,#6579,#3981,.T.);
#8454=EDGE_CURVE('',#6580,#6579,#3982,.T.);
#8455=EDGE_CURVE('',#6580,#6581,#3983,.T.);
#8456=EDGE_CURVE('',#6581,#6582,#3984,.T.);
#8457=EDGE_CURVE('',#6583,#6582,#3985,.T.);
#8458=EDGE_CURVE('',#6583,#6584,#3986,.T.);
#8459=EDGE_CURVE('',#6584,#6585,#3987,.T.);
#8460=EDGE_CURVE('',#6586,#6585,#3988,.T.);
#8461=EDGE_CURVE('',#6586,#6587,#3989,.T.);
#8462=EDGE_CURVE('',#6587,#6588,#3990,.T.);
#8463=EDGE_CURVE('',#6589,#6588,#3991,.T.);
#8464=EDGE_CURVE('',#6589,#6590,#3992,.T.);
#8465=EDGE_CURVE('',#6590,#6591,#3993,.T.);
#8466=EDGE_CURVE('',#6592,#6591,#3994,.T.);
#8467=EDGE_CURVE('',#6592,#6593,#3995,.T.);
#8468=EDGE_CURVE('',#6593,#6594,#3996,.T.);
#8469=EDGE_CURVE('',#6595,#6594,#3997,.T.);
#8470=EDGE_CURVE('',#6595,#6596,#3998,.T.);
#8471=EDGE_CURVE('',#6596,#6597,#3999,.T.);
#8472=EDGE_CURVE('',#6598,#6597,#4000,.T.);
#8473=EDGE_CURVE('',#6598,#6599,#4001,.T.);
#8474=EDGE_CURVE('',#6599,#6600,#4002,.T.);
#8475=EDGE_CURVE('',#6601,#6600,#4003,.T.);
#8476=EDGE_CURVE('',#6601,#6602,#4004,.T.);
#8477=EDGE_CURVE('',#6602,#6603,#4005,.T.);
#8478=EDGE_CURVE('',#6604,#6603,#4006,.T.);
#8479=EDGE_CURVE('',#6604,#6605,#4007,.T.);
#8480=EDGE_CURVE('',#6605,#6606,#4008,.T.);
#8481=EDGE_CURVE('',#6607,#6606,#4009,.T.);
#8482=EDGE_CURVE('',#6607,#6608,#4010,.T.);
#8483=EDGE_CURVE('',#6608,#6609,#4011,.T.);
#8484=EDGE_CURVE('',#6610,#6609,#4012,.T.);
#8485=EDGE_CURVE('',#6610,#6611,#4013,.T.);
#8486=EDGE_CURVE('',#6611,#6612,#4014,.T.);
#8487=EDGE_CURVE('',#6613,#6612,#4015,.T.);
#8488=EDGE_CURVE('',#6613,#6614,#4016,.T.);
#8489=EDGE_CURVE('',#6614,#6615,#4017,.T.);
#8490=EDGE_CURVE('',#6616,#6615,#4018,.T.);
#8491=EDGE_CURVE('',#6616,#6617,#4019,.T.);
#8492=EDGE_CURVE('',#6617,#6618,#4020,.T.);
#8493=EDGE_CURVE('',#6619,#6618,#4021,.T.);
#8494=EDGE_CURVE('',#6619,#6620,#4022,.T.);
#8495=EDGE_CURVE('',#6620,#6621,#4023,.T.);
#8496=EDGE_CURVE('',#6622,#6621,#4024,.T.);
#8497=EDGE_CURVE('',#6622,#6623,#4025,.T.);
#8498=EDGE_CURVE('',#6623,#6624,#4026,.T.);
#8499=EDGE_CURVE('',#6625,#6624,#4027,.T.);
#8500=EDGE_CURVE('',#6625,#6626,#4028,.T.);
#8501=EDGE_CURVE('',#6626,#6627,#4029,.T.);
#8502=EDGE_CURVE('',#6628,#6627,#4030,.T.);
#8503=EDGE_CURVE('',#6628,#6629,#4031,.T.);
#8504=EDGE_CURVE('',#6629,#6630,#4032,.T.);
#8505=EDGE_CURVE('',#6631,#6630,#4033,.T.);
#8506=EDGE_CURVE('',#6631,#6632,#4034,.T.);
#8507=EDGE_CURVE('',#6632,#6633,#4035,.T.);
#8508=EDGE_CURVE('',#6574,#6633,#4036,.T.);
#8509=EDGE_CURVE('',#6633,#6634,#4037,.F.);
#8510=EDGE_CURVE('',#6634,#6635,#4038,.T.);
#8511=EDGE_CURVE('',#6635,#6574,#4039,.F.);
#8512=EDGE_CURVE('',#6636,#6634,#4040,.T.);
#8513=EDGE_CURVE('',#6636,#6637,#4041,.T.);
#8514=EDGE_CURVE('',#6637,#6635,#4042,.T.);
#8515=EDGE_CURVE('',#6579,#6638,#4043,.F.);
#8516=EDGE_CURVE('',#6638,#6639,#4044,.T.);
#8517=EDGE_CURVE('',#6639,#6580,#4045,.F.);
#8518=EDGE_CURVE('',#6640,#6638,#4046,.T.);
#8519=EDGE_CURVE('',#6640,#6641,#4047,.T.);
#8520=EDGE_CURVE('',#6641,#6639,#4048,.T.);
#8521=EDGE_CURVE('',#6585,#6642,#4049,.F.);
#8522=EDGE_CURVE('',#6642,#6643,#4050,.T.);
#8523=EDGE_CURVE('',#6643,#6586,#4051,.F.);
#8524=EDGE_CURVE('',#6644,#6642,#4052,.T.);
#8525=EDGE_CURVE('',#6644,#6645,#4053,.T.);
#8526=EDGE_CURVE('',#6645,#6643,#4054,.T.);
#8527=EDGE_CURVE('',#6646,#6647,#4055,.T.);
#8528=EDGE_CURVE('',#6564,#6646,#4056,.T.);
#8529=EDGE_CURVE('',#6647,#6564,#4057,.T.);
#8530=EDGE_CURVE('',#6648,#6563,#4058,.T.);
#8531=EDGE_CURVE('',#6646,#6649,#4059,.T.);
#8532=EDGE_CURVE('',#6649,#6648,#4060,.T.);
#8533=EDGE_CURVE('',#6650,#6651,#4061,.T.);
#8534=EDGE_CURVE('',#6572,#6650,#4062,.T.);
#8535=EDGE_CURVE('',#6651,#6572,#4063,.T.);
#8536=EDGE_CURVE('',#6650,#6647,#4064,.T.);
#8537=EDGE_CURVE('',#6652,#6653,#4065,.T.);
#8538=EDGE_CURVE('',#6571,#6652,#4066,.T.);
#8539=EDGE_CURVE('',#6653,#6571,#4067,.T.);
#8540=EDGE_CURVE('',#6652,#6651,#4068,.T.);
#8541=EDGE_CURVE('',#6654,#6655,#4069,.T.);
#8542=EDGE_CURVE('',#6655,#6653,#4070,.T.);
#8543=EDGE_CURVE('',#6570,#6654,#4071,.T.);
#8544=EDGE_CURVE('',#6588,#6652,#4072,.T.);
#8545=EDGE_CURVE('',#6653,#6589,#4073,.T.);
#8546=EDGE_CURVE('',#6582,#6650,#4074,.T.);
#8547=EDGE_CURVE('',#6651,#6583,#4075,.T.);
#8548=EDGE_CURVE('',#6576,#6646,#4076,.T.);
#8549=EDGE_CURVE('',#6647,#6577,#4077,.T.);
#8550=EDGE_CURVE('',#6581,#6656,#4078,.T.);
#8551=EDGE_CURVE('',#6656,#6657,#4079,.T.);
#8552=EDGE_CURVE('',#6657,#6578,#4080,.T.);
#8553=EDGE_CURVE('',#6587,#6658,#4081,.T.);
#8554=EDGE_CURVE('',#6658,#6659,#4082,.T.);
#8555=EDGE_CURVE('',#6659,#6584,#4083,.T.);
#8556=EDGE_CURVE('',#6594,#6655,#4084,.T.);
#8557=EDGE_CURVE('',#6593,#6660,#4085,.T.);
#8558=EDGE_CURVE('',#6660,#6661,#4086,.T.);
#8559=EDGE_CURVE('',#6661,#6590,#4087,.T.);
#8560=EDGE_CURVE('',#6662,#6654,#4088,.T.);
#8561=EDGE_CURVE('',#6662,#6595,#4089,.T.);
#8562=EDGE_CURVE('',#6569,#6663,#4090,.T.);
#8563=EDGE_CURVE('',#6663,#6662,#4091,.T.);
#8564=EDGE_CURVE('',#6591,#6664,#4092,.F.);
#8565=EDGE_CURVE('',#6664,#6665,#4093,.T.);
#8566=EDGE_CURVE('',#6665,#6592,#4094,.F.);
#8567=EDGE_CURVE('',#6666,#6664,#4095,.T.);
#8568=EDGE_CURVE('',#6666,#6667,#4096,.T.);
#8569=EDGE_CURVE('',#6667,#6665,#4097,.T.);
#8570=EDGE_CURVE('',#6597,#6668,#4098,.F.);
#8571=EDGE_CURVE('',#6668,#6669,#4099,.T.);
#8572=EDGE_CURVE('',#6669,#6598,#4100,.F.);
#8573=EDGE_CURVE('',#6670,#6668,#4101,.T.);
#8574=EDGE_CURVE('',#6670,#6671,#4102,.T.);
#8575=EDGE_CURVE('',#6671,#6669,#4103,.T.);
#8576=EDGE_CURVE('',#6603,#6672,#4104,.F.);
#8577=EDGE_CURVE('',#6672,#6673,#4105,.T.);
#8578=EDGE_CURVE('',#6673,#6604,#4106,.F.);
#8579=EDGE_CURVE('',#6674,#6672,#4107,.T.);
#8580=EDGE_CURVE('',#6674,#6675,#4108,.T.);
#8581=EDGE_CURVE('',#6675,#6673,#4109,.T.);
#8582=EDGE_CURVE('',#6609,#6676,#4110,.F.);
#8583=EDGE_CURVE('',#6676,#6677,#4111,.T.);
#8584=EDGE_CURVE('',#6677,#6610,#4112,.F.);
#8585=EDGE_CURVE('',#6678,#6676,#4113,.T.);
#8586=EDGE_CURVE('',#6678,#6679,#4114,.T.);
#8587=EDGE_CURVE('',#6679,#6677,#4115,.T.);
#8588=EDGE_CURVE('',#6615,#6680,#4116,.F.);
#8589=EDGE_CURVE('',#6680,#6681,#4117,.T.);
#8590=EDGE_CURVE('',#6681,#6616,#4118,.F.);
#8591=EDGE_CURVE('',#6682,#6680,#4119,.T.);
#8592=EDGE_CURVE('',#6682,#6683,#4120,.T.);
#8593=EDGE_CURVE('',#6683,#6681,#4121,.T.);
#8594=EDGE_CURVE('',#6621,#6684,#4122,.F.);
#8595=EDGE_CURVE('',#6684,#6685,#4123,.T.);
#8596=EDGE_CURVE('',#6685,#6622,#4124,.F.);
#8597=EDGE_CURVE('',#6686,#6684,#4125,.T.);
#8598=EDGE_CURVE('',#6686,#6687,#4126,.T.);
#8599=EDGE_CURVE('',#6687,#6685,#4127,.T.);
#8600=EDGE_CURVE('',#6663,#6688,#4128,.T.);
#8601=EDGE_CURVE('',#6688,#6569,#4129,.T.);
#8602=EDGE_CURVE('',#6689,#6690,#4130,.T.);
#8603=EDGE_CURVE('',#6568,#6689,#4131,.T.);
#8604=EDGE_CURVE('',#6690,#6568,#4132,.T.);
#8605=EDGE_CURVE('',#6689,#6688,#4133,.T.);
#8606=EDGE_CURVE('',#6691,#6692,#4134,.T.);
#8607=EDGE_CURVE('',#6567,#6691,#4135,.T.);
#8608=EDGE_CURVE('',#6692,#6567,#4136,.T.);
#8609=EDGE_CURVE('',#6691,#6690,#4137,.T.);
#8610=EDGE_CURVE('',#6693,#6694,#4138,.T.);
#8611=EDGE_CURVE('',#6566,#6693,#4139,.T.);
#8612=EDGE_CURVE('',#6694,#6566,#4140,.T.);
#8613=EDGE_CURVE('',#6693,#6692,#4141,.T.);
#8614=EDGE_CURVE('',#6565,#6695,#4142,.T.);
#8615=EDGE_CURVE('',#6696,#6565,#4143,.T.);
#8616=EDGE_CURVE('',#6695,#6696,#4144,.T.);
#8617=EDGE_CURVE('',#6648,#6697,#4145,.T.);
#8618=EDGE_CURVE('',#6697,#6696,#4146,.T.);
#8619=EDGE_CURVE('',#6624,#6695,#4147,.T.);
#8620=EDGE_CURVE('',#6696,#6625,#4148,.T.);
#8621=EDGE_CURVE('',#6695,#6694,#4149,.T.);
#8622=EDGE_CURVE('',#6649,#6631,#4150,.T.);
#8623=EDGE_CURVE('',#6630,#6697,#4151,.T.);
#8624=EDGE_CURVE('',#6618,#6693,#4152,.T.);
#8625=EDGE_CURVE('',#6694,#6619,#4153,.T.);
#8626=EDGE_CURVE('',#6612,#6691,#4154,.T.);
#8627=EDGE_CURVE('',#6692,#6613,#4155,.T.);
#8628=EDGE_CURVE('',#6606,#6689,#4156,.T.);
#8629=EDGE_CURVE('',#6690,#6607,#4157,.T.);
#8630=EDGE_CURVE('',#6600,#6663,#4158,.T.);
#8631=EDGE_CURVE('',#6688,#6601,#4159,.T.);
#8632=EDGE_CURVE('',#6599,#6698,#4160,.T.);
#8633=EDGE_CURVE('',#6698,#6699,#4161,.T.);
#8634=EDGE_CURVE('',#6699,#6596,#4162,.T.);
#8635=EDGE_CURVE('',#6605,#6700,#4163,.T.);
#8636=EDGE_CURVE('',#6700,#6701,#4164,.T.);
#8637=EDGE_CURVE('',#6701,#6602,#4165,.T.);
#8638=EDGE_CURVE('',#6611,#6702,#4166,.T.);
#8639=EDGE_CURVE('',#6702,#6703,#4167,.T.);
#8640=EDGE_CURVE('',#6703,#6608,#4168,.T.);
#8641=EDGE_CURVE('',#6617,#6704,#4169,.T.);
#8642=EDGE_CURVE('',#6704,#6705,#4170,.T.);
#8643=EDGE_CURVE('',#6705,#6614,#4171,.T.);
#8644=EDGE_CURVE('',#6623,#6706,#4172,.T.);
#8645=EDGE_CURVE('',#6706,#6707,#4173,.T.);
#8646=EDGE_CURVE('',#6707,#6620,#4174,.T.);
#8647=EDGE_CURVE('',#6627,#6708,#4175,.F.);
#8648=EDGE_CURVE('',#6708,#6709,#4176,.T.);
#8649=EDGE_CURVE('',#6709,#6628,#4177,.F.);
#8650=EDGE_CURVE('',#6710,#6708,#4178,.T.);
#8651=EDGE_CURVE('',#6710,#6711,#4179,.T.);
#8652=EDGE_CURVE('',#6711,#6709,#4180,.T.);
#8653=EDGE_CURVE('',#6712,#6713,#4181,.T.);
#8654=EDGE_CURVE('',#6711,#6712,#4182,.T.);
#8655=EDGE_CURVE('',#6713,#6710,#4183,.T.);
#8656=EDGE_CURVE('',#6713,#6626,#4184,.T.);
#8657=EDGE_CURVE('',#6629,#6712,#4185,.T.);
#8658=EDGE_CURVE('',#6687,#6706,#4186,.T.);
#8659=EDGE_CURVE('',#6707,#6686,#4187,.T.);
#8660=EDGE_CURVE('',#6683,#6704,#4188,.T.);
#8661=EDGE_CURVE('',#6705,#6682,#4189,.T.);
#8662=EDGE_CURVE('',#6679,#6702,#4190,.T.);
#8663=EDGE_CURVE('',#6703,#6678,#4191,.T.);
#8664=EDGE_CURVE('',#6675,#6700,#4192,.T.);
#8665=EDGE_CURVE('',#6701,#6674,#4193,.T.);
#8666=EDGE_CURVE('',#6671,#6698,#4194,.T.);
#8667=EDGE_CURVE('',#6699,#6670,#4195,.T.);
#8668=EDGE_CURVE('',#6667,#6660,#4196,.T.);
#8669=EDGE_CURVE('',#6661,#6666,#4197,.T.);
#8670=EDGE_CURVE('',#6645,#6658,#4198,.T.);
#8671=EDGE_CURVE('',#6659,#6644,#4199,.T.);
#8672=EDGE_CURVE('',#6641,#6656,#4200,.T.);
#8673=EDGE_CURVE('',#6657,#6640,#4201,.T.);
#8674=EDGE_CURVE('',#6714,#6632,#4202,.T.);
#8675=EDGE_CURVE('',#6714,#6636,#4203,.T.);
#8676=EDGE_CURVE('',#6575,#6715,#4204,.T.);
#8677=EDGE_CURVE('',#6637,#6715,#4205,.T.);
#8678=EDGE_CURVE('',#6715,#6714,#4206,.T.);
#12111=ORIENTED_EDGE('',*,*,#8432,.T.);
#12112=ORIENTED_EDGE('',*,*,#8433,.T.);
#12113=ORIENTED_EDGE('',*,*,#8434,.T.);
#12114=ORIENTED_EDGE('',*,*,#8433,.F.);
#12115=ORIENTED_EDGE('',*,*,#8435,.F.);
#12116=ORIENTED_EDGE('',*,*,#8436,.T.);
#12117=ORIENTED_EDGE('',*,*,#8432,.F.);
#12118=ORIENTED_EDGE('',*,*,#8436,.F.);
#12119=ORIENTED_EDGE('',*,*,#8437,.F.);
#12120=ORIENTED_EDGE('',*,*,#8438,.F.);
#12121=ORIENTED_EDGE('',*,*,#8439,.F.);
#12122=ORIENTED_EDGE('',*,*,#8440,.F.);
#12123=ORIENTED_EDGE('',*,*,#8441,.F.);
#12124=ORIENTED_EDGE('',*,*,#8442,.F.);
#12125=ORIENTED_EDGE('',*,*,#8443,.F.);
#12126=ORIENTED_EDGE('',*,*,#8444,.F.);
#12127=ORIENTED_EDGE('',*,*,#8445,.F.);
#12128=ORIENTED_EDGE('',*,*,#8446,.F.);
#12129=ORIENTED_EDGE('',*,*,#8434,.F.);
#12130=ORIENTED_EDGE('',*,*,#8447,.T.);
#12131=ORIENTED_EDGE('',*,*,#8448,.T.);
#12132=ORIENTED_EDGE('',*,*,#8435,.T.);
#12133=ORIENTED_EDGE('',*,*,#8448,.F.);
#12134=ORIENTED_EDGE('',*,*,#8449,.T.);
#12135=ORIENTED_EDGE('',*,*,#8450,.T.);
#12136=ORIENTED_EDGE('',*,*,#8451,.F.);
#12137=ORIENTED_EDGE('',*,*,#8452,.T.);
#12138=ORIENTED_EDGE('',*,*,#8453,.T.);
#12139=ORIENTED_EDGE('',*,*,#8454,.F.);
#12140=ORIENTED_EDGE('',*,*,#8455,.T.);
#12141=ORIENTED_EDGE('',*,*,#8456,.T.);
#12142=ORIENTED_EDGE('',*,*,#8457,.F.);
#12143=ORIENTED_EDGE('',*,*,#8458,.T.);
#12144=ORIENTED_EDGE('',*,*,#8459,.T.);
#12145=ORIENTED_EDGE('',*,*,#8460,.F.);
#12146=ORIENTED_EDGE('',*,*,#8461,.T.);
#12147=ORIENTED_EDGE('',*,*,#8462,.T.);
#12148=ORIENTED_EDGE('',*,*,#8463,.F.);
#12149=ORIENTED_EDGE('',*,*,#8464,.T.);
#12150=ORIENTED_EDGE('',*,*,#8465,.T.);
#12151=ORIENTED_EDGE('',*,*,#8466,.F.);
#12152=ORIENTED_EDGE('',*,*,#8467,.T.);
#12153=ORIENTED_EDGE('',*,*,#8468,.T.);
#12154=ORIENTED_EDGE('',*,*,#8469,.F.);
#12155=ORIENTED_EDGE('',*,*,#8470,.T.);
#12156=ORIENTED_EDGE('',*,*,#8471,.T.);
#12157=ORIENTED_EDGE('',*,*,#8472,.F.);
#12158=ORIENTED_EDGE('',*,*,#8473,.T.);
#12159=ORIENTED_EDGE('',*,*,#8474,.T.);
#12160=ORIENTED_EDGE('',*,*,#8475,.F.);
#12161=ORIENTED_EDGE('',*,*,#8476,.T.);
#12162=ORIENTED_EDGE('',*,*,#8477,.T.);
#12163=ORIENTED_EDGE('',*,*,#8478,.F.);
#12164=ORIENTED_EDGE('',*,*,#8479,.T.);
#12165=ORIENTED_EDGE('',*,*,#8480,.T.);
#12166=ORIENTED_EDGE('',*,*,#8481,.F.);
#12167=ORIENTED_EDGE('',*,*,#8482,.T.);
#12168=ORIENTED_EDGE('',*,*,#8483,.T.);
#12169=ORIENTED_EDGE('',*,*,#8484,.F.);
#12170=ORIENTED_EDGE('',*,*,#8485,.T.);
#12171=ORIENTED_EDGE('',*,*,#8486,.T.);
#12172=ORIENTED_EDGE('',*,*,#8487,.F.);
#12173=ORIENTED_EDGE('',*,*,#8488,.T.);
#12174=ORIENTED_EDGE('',*,*,#8489,.T.);
#12175=ORIENTED_EDGE('',*,*,#8490,.F.);
#12176=ORIENTED_EDGE('',*,*,#8491,.T.);
#12177=ORIENTED_EDGE('',*,*,#8492,.T.);
#12178=ORIENTED_EDGE('',*,*,#8493,.F.);
#12179=ORIENTED_EDGE('',*,*,#8494,.T.);
#12180=ORIENTED_EDGE('',*,*,#8495,.T.);
#12181=ORIENTED_EDGE('',*,*,#8496,.F.);
#12182=ORIENTED_EDGE('',*,*,#8497,.T.);
#12183=ORIENTED_EDGE('',*,*,#8498,.T.);
#12184=ORIENTED_EDGE('',*,*,#8499,.F.);
#12185=ORIENTED_EDGE('',*,*,#8500,.T.);
#12186=ORIENTED_EDGE('',*,*,#8501,.T.);
#12187=ORIENTED_EDGE('',*,*,#8502,.F.);
#12188=ORIENTED_EDGE('',*,*,#8503,.T.);
#12189=ORIENTED_EDGE('',*,*,#8504,.T.);
#12190=ORIENTED_EDGE('',*,*,#8505,.F.);
#12191=ORIENTED_EDGE('',*,*,#8506,.T.);
#12192=ORIENTED_EDGE('',*,*,#8507,.T.);
#12193=ORIENTED_EDGE('',*,*,#8508,.F.);
#12194=ORIENTED_EDGE('',*,*,#8447,.F.);
#12195=ORIENTED_EDGE('',*,*,#8509,.T.);
#12196=ORIENTED_EDGE('',*,*,#8510,.T.);
#12197=ORIENTED_EDGE('',*,*,#8511,.T.);
#12198=ORIENTED_EDGE('',*,*,#8508,.T.);
#12199=ORIENTED_EDGE('',*,*,#8510,.F.);
#12200=ORIENTED_EDGE('',*,*,#8512,.F.);
#12201=ORIENTED_EDGE('',*,*,#8513,.T.);
#12202=ORIENTED_EDGE('',*,*,#8514,.T.);
#12203=ORIENTED_EDGE('',*,*,#8515,.T.);
#12204=ORIENTED_EDGE('',*,*,#8516,.T.);
#12205=ORIENTED_EDGE('',*,*,#8517,.T.);
#12206=ORIENTED_EDGE('',*,*,#8454,.T.);
#12207=ORIENTED_EDGE('',*,*,#8516,.F.);
#12208=ORIENTED_EDGE('',*,*,#8518,.F.);
#12209=ORIENTED_EDGE('',*,*,#8519,.T.);
#12210=ORIENTED_EDGE('',*,*,#8520,.T.);
#12211=ORIENTED_EDGE('',*,*,#8521,.T.);
#12212=ORIENTED_EDGE('',*,*,#8522,.T.);
#12213=ORIENTED_EDGE('',*,*,#8523,.T.);
#12214=ORIENTED_EDGE('',*,*,#8460,.T.);
#12215=ORIENTED_EDGE('',*,*,#8522,.F.);
#12216=ORIENTED_EDGE('',*,*,#8524,.F.);
#12217=ORIENTED_EDGE('',*,*,#8525,.T.);
#12218=ORIENTED_EDGE('',*,*,#8526,.T.);
#12219=ORIENTED_EDGE('',*,*,#8527,.F.);
#12220=ORIENTED_EDGE('',*,*,#8528,.F.);
#12221=ORIENTED_EDGE('',*,*,#8529,.F.);
#12222=ORIENTED_EDGE('',*,*,#8530,.T.);
#12223=ORIENTED_EDGE('',*,*,#8437,.T.);
#12224=ORIENTED_EDGE('',*,*,#8528,.T.);
#12225=ORIENTED_EDGE('',*,*,#8531,.T.);
#12226=ORIENTED_EDGE('',*,*,#8532,.T.);
#12227=ORIENTED_EDGE('',*,*,#8533,.F.);
#12228=ORIENTED_EDGE('',*,*,#8534,.F.);
#12229=ORIENTED_EDGE('',*,*,#8535,.F.);
#12230=ORIENTED_EDGE('',*,*,#8534,.T.);
#12231=ORIENTED_EDGE('',*,*,#8536,.T.);
#12232=ORIENTED_EDGE('',*,*,#8529,.T.);
#12233=ORIENTED_EDGE('',*,*,#8446,.T.);
#12234=ORIENTED_EDGE('',*,*,#8537,.F.);
#12235=ORIENTED_EDGE('',*,*,#8538,.F.);
#12236=ORIENTED_EDGE('',*,*,#8539,.F.);
#12237=ORIENTED_EDGE('',*,*,#8538,.T.);
#12238=ORIENTED_EDGE('',*,*,#8540,.T.);
#12239=ORIENTED_EDGE('',*,*,#8535,.T.);
#12240=ORIENTED_EDGE('',*,*,#8445,.T.);
#12241=ORIENTED_EDGE('',*,*,#8541,.T.);
#12242=ORIENTED_EDGE('',*,*,#8542,.T.);
#12243=ORIENTED_EDGE('',*,*,#8539,.T.);
#12244=ORIENTED_EDGE('',*,*,#8444,.T.);
#12245=ORIENTED_EDGE('',*,*,#8543,.T.);
#12246=ORIENTED_EDGE('',*,*,#8463,.T.);
#12247=ORIENTED_EDGE('',*,*,#8544,.T.);
#12248=ORIENTED_EDGE('',*,*,#8537,.T.);
#12249=ORIENTED_EDGE('',*,*,#8545,.T.);
#12250=ORIENTED_EDGE('',*,*,#8457,.T.);
#12251=ORIENTED_EDGE('',*,*,#8546,.T.);
#12252=ORIENTED_EDGE('',*,*,#8533,.T.);
#12253=ORIENTED_EDGE('',*,*,#8547,.T.);
#12254=ORIENTED_EDGE('',*,*,#8451,.T.);
#12255=ORIENTED_EDGE('',*,*,#8548,.T.);
#12256=ORIENTED_EDGE('',*,*,#8527,.T.);
#12257=ORIENTED_EDGE('',*,*,#8549,.T.);
#12258=ORIENTED_EDGE('',*,*,#8549,.F.);
#12259=ORIENTED_EDGE('',*,*,#8536,.F.);
#12260=ORIENTED_EDGE('',*,*,#8546,.F.);
#12261=ORIENTED_EDGE('',*,*,#8456,.F.);
#12262=ORIENTED_EDGE('',*,*,#8550,.T.);
#12263=ORIENTED_EDGE('',*,*,#8551,.T.);
#12264=ORIENTED_EDGE('',*,*,#8552,.T.);
#12265=ORIENTED_EDGE('',*,*,#8452,.F.);
#12266=ORIENTED_EDGE('',*,*,#8547,.F.);
#12267=ORIENTED_EDGE('',*,*,#8540,.F.);
#12268=ORIENTED_EDGE('',*,*,#8544,.F.);
#12269=ORIENTED_EDGE('',*,*,#8462,.F.);
#12270=ORIENTED_EDGE('',*,*,#8553,.T.);
#12271=ORIENTED_EDGE('',*,*,#8554,.T.);
#12272=ORIENTED_EDGE('',*,*,#8555,.T.);
#12273=ORIENTED_EDGE('',*,*,#8458,.F.);
#12274=ORIENTED_EDGE('',*,*,#8545,.F.);
#12275=ORIENTED_EDGE('',*,*,#8542,.F.);
#12276=ORIENTED_EDGE('',*,*,#8556,.F.);
#12277=ORIENTED_EDGE('',*,*,#8468,.F.);
#12278=ORIENTED_EDGE('',*,*,#8557,.T.);
#12279=ORIENTED_EDGE('',*,*,#8558,.T.);
#12280=ORIENTED_EDGE('',*,*,#8559,.T.);
#12281=ORIENTED_EDGE('',*,*,#8464,.F.);
#12282=ORIENTED_EDGE('',*,*,#8541,.F.);
#12283=ORIENTED_EDGE('',*,*,#8560,.F.);
#12284=ORIENTED_EDGE('',*,*,#8561,.T.);
#12285=ORIENTED_EDGE('',*,*,#8469,.T.);
#12286=ORIENTED_EDGE('',*,*,#8556,.T.);
#12287=ORIENTED_EDGE('',*,*,#8543,.F.);
#12288=ORIENTED_EDGE('',*,*,#8443,.T.);
#12289=ORIENTED_EDGE('',*,*,#8562,.T.);
#12290=ORIENTED_EDGE('',*,*,#8563,.T.);
#12291=ORIENTED_EDGE('',*,*,#8560,.T.);
#12292=ORIENTED_EDGE('',*,*,#8564,.T.);
#12293=ORIENTED_EDGE('',*,*,#8565,.T.);
#12294=ORIENTED_EDGE('',*,*,#8566,.T.);
#12295=ORIENTED_EDGE('',*,*,#8466,.T.);
#12296=ORIENTED_EDGE('',*,*,#8565,.F.);
#12297=ORIENTED_EDGE('',*,*,#8567,.F.);
#12298=ORIENTED_EDGE('',*,*,#8568,.T.);
#12299=ORIENTED_EDGE('',*,*,#8569,.T.);
#12300=ORIENTED_EDGE('',*,*,#8570,.T.);
#12301=ORIENTED_EDGE('',*,*,#8571,.T.);
#12302=ORIENTED_EDGE('',*,*,#8572,.T.);
#12303=ORIENTED_EDGE('',*,*,#8472,.T.);
#12304=ORIENTED_EDGE('',*,*,#8571,.F.);
#12305=ORIENTED_EDGE('',*,*,#8573,.F.);
#12306=ORIENTED_EDGE('',*,*,#8574,.T.);
#12307=ORIENTED_EDGE('',*,*,#8575,.T.);
#12308=ORIENTED_EDGE('',*,*,#8576,.T.);
#12309=ORIENTED_EDGE('',*,*,#8577,.T.);
#12310=ORIENTED_EDGE('',*,*,#8578,.T.);
#12311=ORIENTED_EDGE('',*,*,#8478,.T.);
#12312=ORIENTED_EDGE('',*,*,#8577,.F.);
#12313=ORIENTED_EDGE('',*,*,#8579,.F.);
#12314=ORIENTED_EDGE('',*,*,#8580,.T.);
#12315=ORIENTED_EDGE('',*,*,#8581,.T.);
#12316=ORIENTED_EDGE('',*,*,#8582,.T.);
#12317=ORIENTED_EDGE('',*,*,#8583,.T.);
#12318=ORIENTED_EDGE('',*,*,#8584,.T.);
#12319=ORIENTED_EDGE('',*,*,#8484,.T.);
#12320=ORIENTED_EDGE('',*,*,#8583,.F.);
#12321=ORIENTED_EDGE('',*,*,#8585,.F.);
#12322=ORIENTED_EDGE('',*,*,#8586,.T.);
#12323=ORIENTED_EDGE('',*,*,#8587,.T.);
#12324=ORIENTED_EDGE('',*,*,#8588,.T.);
#12325=ORIENTED_EDGE('',*,*,#8589,.T.);
#12326=ORIENTED_EDGE('',*,*,#8590,.T.);
#12327=ORIENTED_EDGE('',*,*,#8490,.T.);
#12328=ORIENTED_EDGE('',*,*,#8589,.F.);
#12329=ORIENTED_EDGE('',*,*,#8591,.F.);
#12330=ORIENTED_EDGE('',*,*,#8592,.T.);
#12331=ORIENTED_EDGE('',*,*,#8593,.T.);
#12332=ORIENTED_EDGE('',*,*,#8594,.T.);
#12333=ORIENTED_EDGE('',*,*,#8595,.T.);
#12334=ORIENTED_EDGE('',*,*,#8596,.T.);
#12335=ORIENTED_EDGE('',*,*,#8496,.T.);
#12336=ORIENTED_EDGE('',*,*,#8595,.F.);
#12337=ORIENTED_EDGE('',*,*,#8597,.F.);
#12338=ORIENTED_EDGE('',*,*,#8598,.T.);
#12339=ORIENTED_EDGE('',*,*,#8599,.T.);
#12340=ORIENTED_EDGE('',*,*,#8600,.F.);
#12341=ORIENTED_EDGE('',*,*,#8562,.F.);
#12342=ORIENTED_EDGE('',*,*,#8601,.F.);
#12343=ORIENTED_EDGE('',*,*,#8602,.F.);
#12344=ORIENTED_EDGE('',*,*,#8603,.F.);
#12345=ORIENTED_EDGE('',*,*,#8604,.F.);
#12346=ORIENTED_EDGE('',*,*,#8603,.T.);
#12347=ORIENTED_EDGE('',*,*,#8605,.T.);
#12348=ORIENTED_EDGE('',*,*,#8601,.T.);
#12349=ORIENTED_EDGE('',*,*,#8442,.T.);
#12350=ORIENTED_EDGE('',*,*,#8606,.F.);
#12351=ORIENTED_EDGE('',*,*,#8607,.F.);
#12352=ORIENTED_EDGE('',*,*,#8608,.F.);
#12353=ORIENTED_EDGE('',*,*,#8607,.T.);
#12354=ORIENTED_EDGE('',*,*,#8609,.T.);
#12355=ORIENTED_EDGE('',*,*,#8604,.T.);
#12356=ORIENTED_EDGE('',*,*,#8441,.T.);
#12357=ORIENTED_EDGE('',*,*,#8610,.F.);
#12358=ORIENTED_EDGE('',*,*,#8611,.F.);
#12359=ORIENTED_EDGE('',*,*,#8612,.F.);
#12360=ORIENTED_EDGE('',*,*,#8611,.T.);
#12361=ORIENTED_EDGE('',*,*,#8613,.T.);
#12362=ORIENTED_EDGE('',*,*,#8608,.T.);
#12363=ORIENTED_EDGE('',*,*,#8440,.T.);
#12364=ORIENTED_EDGE('',*,*,#8614,.F.);
#12365=ORIENTED_EDGE('',*,*,#8615,.F.);
#12366=ORIENTED_EDGE('',*,*,#8616,.F.);
#12367=ORIENTED_EDGE('',*,*,#8530,.F.);
#12368=ORIENTED_EDGE('',*,*,#8617,.T.);
#12369=ORIENTED_EDGE('',*,*,#8618,.T.);
#12370=ORIENTED_EDGE('',*,*,#8615,.T.);
#12371=ORIENTED_EDGE('',*,*,#8438,.T.);
#12372=ORIENTED_EDGE('',*,*,#8499,.T.);
#12373=ORIENTED_EDGE('',*,*,#8619,.T.);
#12374=ORIENTED_EDGE('',*,*,#8616,.T.);
#12375=ORIENTED_EDGE('',*,*,#8620,.T.);
#12376=ORIENTED_EDGE('',*,*,#8614,.T.);
#12377=ORIENTED_EDGE('',*,*,#8621,.T.);
#12378=ORIENTED_EDGE('',*,*,#8612,.T.);
#12379=ORIENTED_EDGE('',*,*,#8439,.T.);
#12380=ORIENTED_EDGE('',*,*,#8532,.F.);
#12381=ORIENTED_EDGE('',*,*,#8622,.T.);
#12382=ORIENTED_EDGE('',*,*,#8505,.T.);
#12383=ORIENTED_EDGE('',*,*,#8623,.T.);
#12384=ORIENTED_EDGE('',*,*,#8617,.F.);
#12385=ORIENTED_EDGE('',*,*,#8493,.T.);
#12386=ORIENTED_EDGE('',*,*,#8624,.T.);
#12387=ORIENTED_EDGE('',*,*,#8610,.T.);
#12388=ORIENTED_EDGE('',*,*,#8625,.T.);
#12389=ORIENTED_EDGE('',*,*,#8487,.T.);
#12390=ORIENTED_EDGE('',*,*,#8626,.T.);
#12391=ORIENTED_EDGE('',*,*,#8606,.T.);
#12392=ORIENTED_EDGE('',*,*,#8627,.T.);
#12393=ORIENTED_EDGE('',*,*,#8481,.T.);
#12394=ORIENTED_EDGE('',*,*,#8628,.T.);
#12395=ORIENTED_EDGE('',*,*,#8602,.T.);
#12396=ORIENTED_EDGE('',*,*,#8629,.T.);
#12397=ORIENTED_EDGE('',*,*,#8475,.T.);
#12398=ORIENTED_EDGE('',*,*,#8630,.T.);
#12399=ORIENTED_EDGE('',*,*,#8600,.T.);
#12400=ORIENTED_EDGE('',*,*,#8631,.T.);
#12401=ORIENTED_EDGE('',*,*,#8561,.F.);
#12402=ORIENTED_EDGE('',*,*,#8563,.F.);
#12403=ORIENTED_EDGE('',*,*,#8630,.F.);
#12404=ORIENTED_EDGE('',*,*,#8474,.F.);
#12405=ORIENTED_EDGE('',*,*,#8632,.T.);
#12406=ORIENTED_EDGE('',*,*,#8633,.T.);
#12407=ORIENTED_EDGE('',*,*,#8634,.T.);
#12408=ORIENTED_EDGE('',*,*,#8470,.F.);
#12409=ORIENTED_EDGE('',*,*,#8631,.F.);
#12410=ORIENTED_EDGE('',*,*,#8605,.F.);
#12411=ORIENTED_EDGE('',*,*,#8628,.F.);
#12412=ORIENTED_EDGE('',*,*,#8480,.F.);
#12413=ORIENTED_EDGE('',*,*,#8635,.T.);
#12414=ORIENTED_EDGE('',*,*,#8636,.T.);
#12415=ORIENTED_EDGE('',*,*,#8637,.T.);
#12416=ORIENTED_EDGE('',*,*,#8476,.F.);
#12417=ORIENTED_EDGE('',*,*,#8629,.F.);
#12418=ORIENTED_EDGE('',*,*,#8609,.F.);
#12419=ORIENTED_EDGE('',*,*,#8626,.F.);
#12420=ORIENTED_EDGE('',*,*,#8486,.F.);
#12421=ORIENTED_EDGE('',*,*,#8638,.T.);
#12422=ORIENTED_EDGE('',*,*,#8639,.T.);
#12423=ORIENTED_EDGE('',*,*,#8640,.T.);
#12424=ORIENTED_EDGE('',*,*,#8482,.F.);
#12425=ORIENTED_EDGE('',*,*,#8627,.F.);
#12426=ORIENTED_EDGE('',*,*,#8613,.F.);
#12427=ORIENTED_EDGE('',*,*,#8624,.F.);
#12428=ORIENTED_EDGE('',*,*,#8492,.F.);
#12429=ORIENTED_EDGE('',*,*,#8641,.T.);
#12430=ORIENTED_EDGE('',*,*,#8642,.T.);
#12431=ORIENTED_EDGE('',*,*,#8643,.T.);
#12432=ORIENTED_EDGE('',*,*,#8488,.F.);
#12433=ORIENTED_EDGE('',*,*,#8625,.F.);
#12434=ORIENTED_EDGE('',*,*,#8621,.F.);
#12435=ORIENTED_EDGE('',*,*,#8619,.F.);
#12436=ORIENTED_EDGE('',*,*,#8498,.F.);
#12437=ORIENTED_EDGE('',*,*,#8644,.T.);
#12438=ORIENTED_EDGE('',*,*,#8645,.T.);
#12439=ORIENTED_EDGE('',*,*,#8646,.T.);
#12440=ORIENTED_EDGE('',*,*,#8494,.F.);
#12441=ORIENTED_EDGE('',*,*,#8647,.T.);
#12442=ORIENTED_EDGE('',*,*,#8648,.T.);
#12443=ORIENTED_EDGE('',*,*,#8649,.T.);
#12444=ORIENTED_EDGE('',*,*,#8502,.T.);
#12445=ORIENTED_EDGE('',*,*,#8648,.F.);
#12446=ORIENTED_EDGE('',*,*,#8650,.F.);
#12447=ORIENTED_EDGE('',*,*,#8651,.T.);
#12448=ORIENTED_EDGE('',*,*,#8652,.T.);
#12449=ORIENTED_EDGE('',*,*,#8653,.F.);
#12450=ORIENTED_EDGE('',*,*,#8654,.F.);
#12451=ORIENTED_EDGE('',*,*,#8651,.F.);
#12452=ORIENTED_EDGE('',*,*,#8655,.F.);
#12453=ORIENTED_EDGE('',*,*,#8656,.F.);
#12454=ORIENTED_EDGE('',*,*,#8655,.T.);
#12455=ORIENTED_EDGE('',*,*,#8650,.T.);
#12456=ORIENTED_EDGE('',*,*,#8647,.F.);
#12457=ORIENTED_EDGE('',*,*,#8501,.F.);
#12458=ORIENTED_EDGE('',*,*,#8657,.F.);
#12459=ORIENTED_EDGE('',*,*,#8503,.F.);
#12460=ORIENTED_EDGE('',*,*,#8649,.F.);
#12461=ORIENTED_EDGE('',*,*,#8652,.F.);
#12462=ORIENTED_EDGE('',*,*,#8654,.T.);
#12463=ORIENTED_EDGE('',*,*,#8623,.F.);
#12464=ORIENTED_EDGE('',*,*,#8504,.F.);
#12465=ORIENTED_EDGE('',*,*,#8657,.T.);
#12466=ORIENTED_EDGE('',*,*,#8653,.T.);
#12467=ORIENTED_EDGE('',*,*,#8656,.T.);
#12468=ORIENTED_EDGE('',*,*,#8500,.F.);
#12469=ORIENTED_EDGE('',*,*,#8620,.F.);
#12470=ORIENTED_EDGE('',*,*,#8618,.F.);
#12471=ORIENTED_EDGE('',*,*,#8645,.F.);
#12472=ORIENTED_EDGE('',*,*,#8658,.F.);
#12473=ORIENTED_EDGE('',*,*,#8598,.F.);
#12474=ORIENTED_EDGE('',*,*,#8659,.F.);
#12475=ORIENTED_EDGE('',*,*,#8646,.F.);
#12476=ORIENTED_EDGE('',*,*,#8659,.T.);
#12477=ORIENTED_EDGE('',*,*,#8597,.T.);
#12478=ORIENTED_EDGE('',*,*,#8594,.F.);
#12479=ORIENTED_EDGE('',*,*,#8495,.F.);
#12480=ORIENTED_EDGE('',*,*,#8644,.F.);
#12481=ORIENTED_EDGE('',*,*,#8497,.F.);
#12482=ORIENTED_EDGE('',*,*,#8596,.F.);
#12483=ORIENTED_EDGE('',*,*,#8599,.F.);
#12484=ORIENTED_EDGE('',*,*,#8658,.T.);
#12485=ORIENTED_EDGE('',*,*,#8642,.F.);
#12486=ORIENTED_EDGE('',*,*,#8660,.F.);
#12487=ORIENTED_EDGE('',*,*,#8592,.F.);
#12488=ORIENTED_EDGE('',*,*,#8661,.F.);
#12489=ORIENTED_EDGE('',*,*,#8643,.F.);
#12490=ORIENTED_EDGE('',*,*,#8661,.T.);
#12491=ORIENTED_EDGE('',*,*,#8591,.T.);
#12492=ORIENTED_EDGE('',*,*,#8588,.F.);
#12493=ORIENTED_EDGE('',*,*,#8489,.F.);
#12494=ORIENTED_EDGE('',*,*,#8641,.F.);
#12495=ORIENTED_EDGE('',*,*,#8491,.F.);
#12496=ORIENTED_EDGE('',*,*,#8590,.F.);
#12497=ORIENTED_EDGE('',*,*,#8593,.F.);
#12498=ORIENTED_EDGE('',*,*,#8660,.T.);
#12499=ORIENTED_EDGE('',*,*,#8639,.F.);
#12500=ORIENTED_EDGE('',*,*,#8662,.F.);
#12501=ORIENTED_EDGE('',*,*,#8586,.F.);
#12502=ORIENTED_EDGE('',*,*,#8663,.F.);
#12503=ORIENTED_EDGE('',*,*,#8640,.F.);
#12504=ORIENTED_EDGE('',*,*,#8663,.T.);
#12505=ORIENTED_EDGE('',*,*,#8585,.T.);
#12506=ORIENTED_EDGE('',*,*,#8582,.F.);
#12507=ORIENTED_EDGE('',*,*,#8483,.F.);
#12508=ORIENTED_EDGE('',*,*,#8638,.F.);
#12509=ORIENTED_EDGE('',*,*,#8485,.F.);
#12510=ORIENTED_EDGE('',*,*,#8584,.F.);
#12511=ORIENTED_EDGE('',*,*,#8587,.F.);
#12512=ORIENTED_EDGE('',*,*,#8662,.T.);
#12513=ORIENTED_EDGE('',*,*,#8636,.F.);
#12514=ORIENTED_EDGE('',*,*,#8664,.F.);
#12515=ORIENTED_EDGE('',*,*,#8580,.F.);
#12516=ORIENTED_EDGE('',*,*,#8665,.F.);
#12517=ORIENTED_EDGE('',*,*,#8637,.F.);
#12518=ORIENTED_EDGE('',*,*,#8665,.T.);
#12519=ORIENTED_EDGE('',*,*,#8579,.T.);
#12520=ORIENTED_EDGE('',*,*,#8576,.F.);
#12521=ORIENTED_EDGE('',*,*,#8477,.F.);
#12522=ORIENTED_EDGE('',*,*,#8635,.F.);
#12523=ORIENTED_EDGE('',*,*,#8479,.F.);
#12524=ORIENTED_EDGE('',*,*,#8578,.F.);
#12525=ORIENTED_EDGE('',*,*,#8581,.F.);
#12526=ORIENTED_EDGE('',*,*,#8664,.T.);
#12527=ORIENTED_EDGE('',*,*,#8633,.F.);
#12528=ORIENTED_EDGE('',*,*,#8666,.F.);
#12529=ORIENTED_EDGE('',*,*,#8574,.F.);
#12530=ORIENTED_EDGE('',*,*,#8667,.F.);
#12531=ORIENTED_EDGE('',*,*,#8634,.F.);
#12532=ORIENTED_EDGE('',*,*,#8667,.T.);
#12533=ORIENTED_EDGE('',*,*,#8573,.T.);
#12534=ORIENTED_EDGE('',*,*,#8570,.F.);
#12535=ORIENTED_EDGE('',*,*,#8471,.F.);
#12536=ORIENTED_EDGE('',*,*,#8632,.F.);
#12537=ORIENTED_EDGE('',*,*,#8473,.F.);
#12538=ORIENTED_EDGE('',*,*,#8572,.F.);
#12539=ORIENTED_EDGE('',*,*,#8575,.F.);
#12540=ORIENTED_EDGE('',*,*,#8666,.T.);
#12541=ORIENTED_EDGE('',*,*,#8558,.F.);
#12542=ORIENTED_EDGE('',*,*,#8668,.F.);
#12543=ORIENTED_EDGE('',*,*,#8568,.F.);
#12544=ORIENTED_EDGE('',*,*,#8669,.F.);
#12545=ORIENTED_EDGE('',*,*,#8559,.F.);
#12546=ORIENTED_EDGE('',*,*,#8669,.T.);
#12547=ORIENTED_EDGE('',*,*,#8567,.T.);
#12548=ORIENTED_EDGE('',*,*,#8564,.F.);
#12549=ORIENTED_EDGE('',*,*,#8465,.F.);
#12550=ORIENTED_EDGE('',*,*,#8557,.F.);
#12551=ORIENTED_EDGE('',*,*,#8467,.F.);
#12552=ORIENTED_EDGE('',*,*,#8566,.F.);
#12553=ORIENTED_EDGE('',*,*,#8569,.F.);
#12554=ORIENTED_EDGE('',*,*,#8668,.T.);
#12555=ORIENTED_EDGE('',*,*,#8554,.F.);
#12556=ORIENTED_EDGE('',*,*,#8670,.F.);
#12557=ORIENTED_EDGE('',*,*,#8525,.F.);
#12558=ORIENTED_EDGE('',*,*,#8671,.F.);
#12559=ORIENTED_EDGE('',*,*,#8555,.F.);
#12560=ORIENTED_EDGE('',*,*,#8671,.T.);
#12561=ORIENTED_EDGE('',*,*,#8524,.T.);
#12562=ORIENTED_EDGE('',*,*,#8521,.F.);
#12563=ORIENTED_EDGE('',*,*,#8459,.F.);
#12564=ORIENTED_EDGE('',*,*,#8553,.F.);
#12565=ORIENTED_EDGE('',*,*,#8461,.F.);
#12566=ORIENTED_EDGE('',*,*,#8523,.F.);
#12567=ORIENTED_EDGE('',*,*,#8526,.F.);
#12568=ORIENTED_EDGE('',*,*,#8670,.T.);
#12569=ORIENTED_EDGE('',*,*,#8551,.F.);
#12570=ORIENTED_EDGE('',*,*,#8672,.F.);
#12571=ORIENTED_EDGE('',*,*,#8519,.F.);
#12572=ORIENTED_EDGE('',*,*,#8673,.F.);
#12573=ORIENTED_EDGE('',*,*,#8552,.F.);
#12574=ORIENTED_EDGE('',*,*,#8673,.T.);
#12575=ORIENTED_EDGE('',*,*,#8518,.T.);
#12576=ORIENTED_EDGE('',*,*,#8515,.F.);
#12577=ORIENTED_EDGE('',*,*,#8453,.F.);
#12578=ORIENTED_EDGE('',*,*,#8550,.F.);
#12579=ORIENTED_EDGE('',*,*,#8455,.F.);
#12580=ORIENTED_EDGE('',*,*,#8517,.F.);
#12581=ORIENTED_EDGE('',*,*,#8520,.F.);
#12582=ORIENTED_EDGE('',*,*,#8672,.T.);
#12583=ORIENTED_EDGE('',*,*,#8674,.F.);
#12584=ORIENTED_EDGE('',*,*,#8675,.T.);
#12585=ORIENTED_EDGE('',*,*,#8512,.T.);
#12586=ORIENTED_EDGE('',*,*,#8509,.F.);
#12587=ORIENTED_EDGE('',*,*,#8507,.F.);
#12588=ORIENTED_EDGE('',*,*,#8676,.F.);
#12589=ORIENTED_EDGE('',*,*,#8449,.F.);
#12590=ORIENTED_EDGE('',*,*,#8511,.F.);
#12591=ORIENTED_EDGE('',*,*,#8514,.F.);
#12592=ORIENTED_EDGE('',*,*,#8677,.T.);
#12593=ORIENTED_EDGE('',*,*,#8678,.F.);
#12594=ORIENTED_EDGE('',*,*,#8677,.F.);
#12595=ORIENTED_EDGE('',*,*,#8513,.F.);
#12596=ORIENTED_EDGE('',*,*,#8675,.F.);
#12597=ORIENTED_EDGE('',*,*,#8548,.F.);
#12598=ORIENTED_EDGE('',*,*,#8450,.F.);
#12599=ORIENTED_EDGE('',*,*,#8676,.T.);
#12600=ORIENTED_EDGE('',*,*,#8678,.T.);
#12601=ORIENTED_EDGE('',*,*,#8674,.T.);
#12602=ORIENTED_EDGE('',*,*,#8506,.F.);
#12603=ORIENTED_EDGE('',*,*,#8622,.F.);
#12604=ORIENTED_EDGE('',*,*,#8531,.F.);
#12915=PLANE('',#14895);
#12916=PLANE('',#14898);
#12917=PLANE('',#14899);
#12918=PLANE('',#14900);
#12919=PLANE('',#14901);
#12920=PLANE('',#14902);
#12921=PLANE('',#14903);
#12922=PLANE('',#14904);
#12923=PLANE('',#14905);
#12924=PLANE('',#14906);
#12925=PLANE('',#14907);
#12926=PLANE('',#14908);
#12927=PLANE('',#14909);
#12928=PLANE('',#14910);
#12929=PLANE('',#14911);
#12930=PLANE('',#14912);
#12931=PLANE('',#14913);
#12932=PLANE('',#14914);
#12933=PLANE('',#14915);
#12934=PLANE('',#14916);
#12935=PLANE('',#14917);
#12936=PLANE('',#14918);
#12937=PLANE('',#14919);
#12938=PLANE('',#14920);
#12939=PLANE('',#14921);
#12940=PLANE('',#14922);
#12941=PLANE('',#14923);
#12942=PLANE('',#14924);
#12943=PLANE('',#14925);
#12944=PLANE('',#14926);
#12945=PLANE('',#14927);
#12946=PLANE('',#14928);
#12947=PLANE('',#14929);
#12948=PLANE('',#14930);
#12949=PLANE('',#14931);
#12950=PLANE('',#14932);
#12951=PLANE('',#14933);
#12952=PLANE('',#14934);
#12953=PLANE('',#14935);
#12954=PLANE('',#14936);
#12955=PLANE('',#14937);
#12956=PLANE('',#14938);
#12957=PLANE('',#14939);
#12958=PLANE('',#14940);
#12959=PLANE('',#14941);
#12960=PLANE('',#14942);
#12961=PLANE('',#14943);
#12962=PLANE('',#14944);
#12963=PLANE('',#14945);
#12964=PLANE('',#14946);
#12965=PLANE('',#14947);
#12966=PLANE('',#14948);
#12967=PLANE('',#14949);
#12968=PLANE('',#14950);
#12969=PLANE('',#14951);
#12970=PLANE('',#14952);
#12971=PLANE('',#14953);
#12972=PLANE('',#14954);
#12973=PLANE('',#14955);
#12974=PLANE('',#14956);
#12975=PLANE('',#14957);
#12976=PLANE('',#14958);
#12977=PLANE('',#14959);
#12978=PLANE('',#14960);
#12979=PLANE('',#14961);
#12980=PLANE('',#14962);
#12981=PLANE('',#14963);
#12982=PLANE('',#14964);
#12983=PLANE('',#14965);
#12984=PLANE('',#14966);
#12985=PLANE('',#14967);
#12986=PLANE('',#14968);
#12987=PLANE('',#14969);
#12988=PLANE('',#14970);
#12989=PLANE('',#14971);
#12990=PLANE('',#14972);
#12991=PLANE('',#14973);
#12992=PLANE('',#14974);
#12993=PLANE('',#14975);
#12994=PLANE('',#14976);
#12995=PLANE('',#14977);
#12996=PLANE('',#14978);
#12997=PLANE('',#14979);
#12998=PLANE('',#14980);
#12999=PLANE('',#14981);
#13000=PLANE('',#14982);
#13001=PLANE('',#14983);
#13002=PLANE('',#14984);
#13003=PLANE('',#14985);
#13004=PLANE('',#14986);
#13711=ADVANCED_FACE('',(#1948),#1240,.F.);
#13712=ADVANCED_FACE('',(#1949),#772,.F.);
#13713=ADVANCED_FACE('',(#1950,#645),#12915,.F.);
#13714=ADVANCED_FACE('',(#1951),#1241,.F.);
#13715=ADVANCED_FACE('',(#1952,#646),#12916,.T.);
#13716=ADVANCED_FACE('',(#1953),#12917,.T.);
#13717=ADVANCED_FACE('',(#1954),#12918,.F.);
#13718=ADVANCED_FACE('',(#1955),#12919,.T.);
#13719=ADVANCED_FACE('',(#1956),#12920,.F.);
#13720=ADVANCED_FACE('',(#1957),#12921,.T.);
#13721=ADVANCED_FACE('',(#1958),#12922,.F.);
#13722=ADVANCED_FACE('',(#1959),#12923,.T.);
#13723=ADVANCED_FACE('',(#1960),#12924,.T.);
#13724=ADVANCED_FACE('',(#1961),#12925,.T.);
#13725=ADVANCED_FACE('',(#1962),#12926,.T.);
#13726=ADVANCED_FACE('',(#1963),#12927,.T.);
#13727=ADVANCED_FACE('',(#1964),#12928,.T.);
#13728=ADVANCED_FACE('',(#1965),#12929,.T.);
#13729=ADVANCED_FACE('',(#1966),#12930,.T.);
#13730=ADVANCED_FACE('',(#1967),#12931,.T.);
#13731=ADVANCED_FACE('',(#1968),#12932,.T.);
#13732=ADVANCED_FACE('',(#1969),#12933,.T.);
#13733=ADVANCED_FACE('',(#1970),#12934,.T.);
#13734=ADVANCED_FACE('',(#1971),#12935,.T.);
#13735=ADVANCED_FACE('',(#1972),#12936,.T.);
#13736=ADVANCED_FACE('',(#1973),#12937,.T.);
#13737=ADVANCED_FACE('',(#1974),#12938,.T.);
#13738=ADVANCED_FACE('',(#1975),#12939,.F.);
#13739=ADVANCED_FACE('',(#1976),#12940,.T.);
#13740=ADVANCED_FACE('',(#1977),#12941,.F.);
#13741=ADVANCED_FACE('',(#1978),#12942,.T.);
#13742=ADVANCED_FACE('',(#1979),#12943,.F.);
#13743=ADVANCED_FACE('',(#1980),#12944,.T.);
#13744=ADVANCED_FACE('',(#1981),#12945,.F.);
#13745=ADVANCED_FACE('',(#1982),#12946,.T.);
#13746=ADVANCED_FACE('',(#1983),#12947,.F.);
#13747=ADVANCED_FACE('',(#1984),#12948,.T.);
#13748=ADVANCED_FACE('',(#1985),#12949,.F.);
#13749=ADVANCED_FACE('',(#1986),#12950,.T.);
#13750=ADVANCED_FACE('',(#1987),#12951,.T.);
#13751=ADVANCED_FACE('',(#1988),#12952,.T.);
#13752=ADVANCED_FACE('',(#1989),#12953,.T.);
#13753=ADVANCED_FACE('',(#1990),#12954,.T.);
#13754=ADVANCED_FACE('',(#1991),#12955,.T.);
#13755=ADVANCED_FACE('',(#1992),#12956,.T.);
#13756=ADVANCED_FACE('',(#1993),#12957,.T.);
#13757=ADVANCED_FACE('',(#1994),#12958,.T.);
#13758=ADVANCED_FACE('',(#1995),#12959,.T.);
#13759=ADVANCED_FACE('',(#1996),#12960,.T.);
#13760=ADVANCED_FACE('',(#1997),#12961,.T.);
#13761=ADVANCED_FACE('',(#1998),#12962,.T.);
#13762=ADVANCED_FACE('',(#1999),#12963,.T.);
#13763=ADVANCED_FACE('',(#2000),#12964,.T.);
#13764=ADVANCED_FACE('',(#2001),#12965,.T.);
#13765=ADVANCED_FACE('',(#2002),#12966,.T.);
#13766=ADVANCED_FACE('',(#2003),#12967,.T.);
#13767=ADVANCED_FACE('',(#2004),#12968,.T.);
#13768=ADVANCED_FACE('',(#2005),#12969,.T.);
#13769=ADVANCED_FACE('',(#2006),#12970,.T.);
#13770=ADVANCED_FACE('',(#2007),#12971,.T.);
#13771=ADVANCED_FACE('',(#2008),#12972,.F.);
#13772=ADVANCED_FACE('',(#2009),#12973,.T.);
#13773=ADVANCED_FACE('',(#2010),#12974,.F.);
#13774=ADVANCED_FACE('',(#2011),#12975,.F.);
#13775=ADVANCED_FACE('',(#2012),#12976,.T.);
#13776=ADVANCED_FACE('',(#2013),#12977,.T.);
#13777=ADVANCED_FACE('',(#2014),#12978,.F.);
#13778=ADVANCED_FACE('',(#2015),#12979,.F.);
#13779=ADVANCED_FACE('',(#2016),#12980,.T.);
#13780=ADVANCED_FACE('',(#2017),#12981,.F.);
#13781=ADVANCED_FACE('',(#2018),#12982,.F.);
#13782=ADVANCED_FACE('',(#2019),#12983,.T.);
#13783=ADVANCED_FACE('',(#2020),#12984,.F.);
#13784=ADVANCED_FACE('',(#2021),#12985,.F.);
#13785=ADVANCED_FACE('',(#2022),#12986,.T.);
#13786=ADVANCED_FACE('',(#2023),#12987,.F.);
#13787=ADVANCED_FACE('',(#2024),#12988,.F.);
#13788=ADVANCED_FACE('',(#2025),#12989,.T.);
#13789=ADVANCED_FACE('',(#2026),#12990,.F.);
#13790=ADVANCED_FACE('',(#2027),#12991,.F.);
#13791=ADVANCED_FACE('',(#2028),#12992,.T.);
#13792=ADVANCED_FACE('',(#2029),#12993,.F.);
#13793=ADVANCED_FACE('',(#2030),#12994,.F.);
#13794=ADVANCED_FACE('',(#2031),#12995,.T.);
#13795=ADVANCED_FACE('',(#2032),#12996,.F.);
#13796=ADVANCED_FACE('',(#2033),#12997,.F.);
#13797=ADVANCED_FACE('',(#2034),#12998,.T.);
#13798=ADVANCED_FACE('',(#2035),#12999,.F.);
#13799=ADVANCED_FACE('',(#2036),#13000,.F.);
#13800=ADVANCED_FACE('',(#2037),#13001,.F.);
#13801=ADVANCED_FACE('',(#2038),#13002,.F.);
#13802=ADVANCED_FACE('',(#2039),#13003,.T.);
#13803=ADVANCED_FACE('',(#2040),#13004,.T.);
#13817=CLOSED_SHELL('',(#13711,#13712,#13713,#13714,#13715,#13716,#13717,
#13718,#13719,#13720,#13721,#13722,#13723,#13724,#13725,#13726,#13727,#13728,
#13729,#13730,#13731,#13732,#13733,#13734,#13735,#13736,#13737,#13738,#13739,
#13740,#13741,#13742,#13743,#13744,#13745,#13746,#13747,#13748,#13749,#13750,
#13751,#13752,#13753,#13754,#13755,#13756,#13757,#13758,#13759,#13760,#13761,
#13762,#13763,#13764,#13765,#13766,#13767,#13768,#13769,#13770,#13771,#13772,
#13773,#13774,#13775,#13776,#13777,#13778,#13779,#13780,#13781,#13782,#13783,
#13784,#13785,#13786,#13787,#13788,#13789,#13790,#13791,#13792,#13793,#13794,
#13795,#13796,#13797,#13798,#13799,#13800,#13801,#13802,#13803));
#14889=AXIS2_PLACEMENT_3D('',#31764,#17904,#17905);
#14890=AXIS2_PLACEMENT_3D('',#31765,#17906,#17907);
#14891=AXIS2_PLACEMENT_3D('',#31767,#17908,#17909);
#14892=AXIS2_PLACEMENT_3D('',#31770,#17911,#17912);
#14893=AXIS2_PLACEMENT_3D('',#31771,#17913,#17914);
#14894=AXIS2_PLACEMENT_3D('',#31773,#17915,#17916);
#14895=AXIS2_PLACEMENT_3D('',#31775,#17918,#17919);
#14896=AXIS2_PLACEMENT_3D('',#31796,#17930,#17931);
#14897=AXIS2_PLACEMENT_3D('',#31798,#17932,#17933);
#14898=AXIS2_PLACEMENT_3D('',#31800,#17935,#17936);
#14899=AXIS2_PLACEMENT_3D('',#31921,#17997,#17998);
#14900=AXIS2_PLACEMENT_3D('',#31927,#18002,#18003);
#14901=AXIS2_PLACEMENT_3D('',#31933,#18007,#18008);
#14902=AXIS2_PLACEMENT_3D('',#31939,#18012,#18013);
#14903=AXIS2_PLACEMENT_3D('',#31945,#18017,#18018);
#14904=AXIS2_PLACEMENT_3D('',#31951,#18022,#18023);
#14905=AXIS2_PLACEMENT_3D('',#31957,#18027,#18028);
#14906=AXIS2_PLACEMENT_3D('',#31963,#18032,#18033);
#14907=AXIS2_PLACEMENT_3D('',#31969,#18037,#18038);
#14908=AXIS2_PLACEMENT_3D('',#31975,#18042,#18043);
#14909=AXIS2_PLACEMENT_3D('',#31977,#18045,#18046);
#14910=AXIS2_PLACEMENT_3D('',#31983,#18050,#18051);
#14911=AXIS2_PLACEMENT_3D('',#31985,#18053,#18054);
#14912=AXIS2_PLACEMENT_3D('',#31991,#18058,#18059);
#14913=AXIS2_PLACEMENT_3D('',#31994,#18062,#18063);
#14914=AXIS2_PLACEMENT_3D('',#31997,#18066,#18067);
#14915=AXIS2_PLACEMENT_3D('',#32000,#18070,#18071);
#14916=AXIS2_PLACEMENT_3D('',#32006,#18075,#18076);
#14917=AXIS2_PLACEMENT_3D('',#32012,#18080,#18081);
#14918=AXIS2_PLACEMENT_3D('',#32019,#18086,#18087);
#14919=AXIS2_PLACEMENT_3D('',#32023,#18090,#18091);
#14920=AXIS2_PLACEMENT_3D('',#32027,#18094,#18095);
#14921=AXIS2_PLACEMENT_3D('',#32033,#18099,#18100);
#14922=AXIS2_PLACEMENT_3D('',#32039,#18104,#18105);
#14923=AXIS2_PLACEMENT_3D('',#32045,#18109,#18110);
#14924=AXIS2_PLACEMENT_3D('',#32051,#18114,#18115);
#14925=AXIS2_PLACEMENT_3D('',#32057,#18119,#18120);
#14926=AXIS2_PLACEMENT_3D('',#32063,#18124,#18125);
#14927=AXIS2_PLACEMENT_3D('',#32069,#18129,#18130);
#14928=AXIS2_PLACEMENT_3D('',#32075,#18134,#18135);
#14929=AXIS2_PLACEMENT_3D('',#32081,#18139,#18140);
#14930=AXIS2_PLACEMENT_3D('',#32087,#18144,#18145);
#14931=AXIS2_PLACEMENT_3D('',#32093,#18149,#18150);
#14932=AXIS2_PLACEMENT_3D('',#32099,#18154,#18155);
#14933=AXIS2_PLACEMENT_3D('',#32103,#18158,#18159);
#14934=AXIS2_PLACEMENT_3D('',#32109,#18163,#18164);
#14935=AXIS2_PLACEMENT_3D('',#32111,#18166,#18167);
#14936=AXIS2_PLACEMENT_3D('',#32117,#18171,#18172);
#14937=AXIS2_PLACEMENT_3D('',#32119,#18174,#18175);
#14938=AXIS2_PLACEMENT_3D('',#32125,#18179,#18180);
#14939=AXIS2_PLACEMENT_3D('',#32127,#18182,#18183);
#14940=AXIS2_PLACEMENT_3D('',#32133,#18187,#18188);
#14941=AXIS2_PLACEMENT_3D('',#32137,#18191,#18192);
#14942=AXIS2_PLACEMENT_3D('',#32140,#18195,#18196);
#14943=AXIS2_PLACEMENT_3D('',#32142,#18198,#18199);
#14944=AXIS2_PLACEMENT_3D('',#32145,#18202,#18203);
#14945=AXIS2_PLACEMENT_3D('',#32148,#18206,#18207);
#14946=AXIS2_PLACEMENT_3D('',#32151,#18210,#18211);
#14947=AXIS2_PLACEMENT_3D('',#32154,#18214,#18215);
#14948=AXIS2_PLACEMENT_3D('',#32157,#18218,#18219);
#14949=AXIS2_PLACEMENT_3D('',#32163,#18223,#18224);
#14950=AXIS2_PLACEMENT_3D('',#32169,#18228,#18229);
#14951=AXIS2_PLACEMENT_3D('',#32175,#18233,#18234);
#14952=AXIS2_PLACEMENT_3D('',#32181,#18238,#18239);
#14953=AXIS2_PLACEMENT_3D('',#32187,#18243,#18244);
#14954=AXIS2_PLACEMENT_3D('',#32193,#18248,#18249);
#14955=AXIS2_PLACEMENT_3D('',#32199,#18253,#18254);
#14956=AXIS2_PLACEMENT_3D('',#32205,#18258,#18259);
#14957=AXIS2_PLACEMENT_3D('',#32207,#18261,#18262);
#14958=AXIS2_PLACEMENT_3D('',#32209,#18264,#18265);
#14959=AXIS2_PLACEMENT_3D('',#32210,#18266,#18267);
#14960=AXIS2_PLACEMENT_3D('',#32213,#18270,#18271);
#14961=AXIS2_PLACEMENT_3D('',#32214,#18272,#18273);
#14962=AXIS2_PLACEMENT_3D('',#32215,#18274,#18275);
#14963=AXIS2_PLACEMENT_3D('',#32218,#18278,#18279);
#14964=AXIS2_PLACEMENT_3D('',#32219,#18280,#18281);
#14965=AXIS2_PLACEMENT_3D('',#32220,#18282,#18283);
#14966=AXIS2_PLACEMENT_3D('',#32223,#18286,#18287);
#14967=AXIS2_PLACEMENT_3D('',#32224,#18288,#18289);
#14968=AXIS2_PLACEMENT_3D('',#32225,#18290,#18291);
#14969=AXIS2_PLACEMENT_3D('',#32228,#18294,#18295);
#14970=AXIS2_PLACEMENT_3D('',#32229,#18296,#18297);
#14971=AXIS2_PLACEMENT_3D('',#32230,#18298,#18299);
#14972=AXIS2_PLACEMENT_3D('',#32233,#18302,#18303);
#14973=AXIS2_PLACEMENT_3D('',#32234,#18304,#18305);
#14974=AXIS2_PLACEMENT_3D('',#32235,#18306,#18307);
#14975=AXIS2_PLACEMENT_3D('',#32238,#18310,#18311);
#14976=AXIS2_PLACEMENT_3D('',#32239,#18312,#18313);
#14977=AXIS2_PLACEMENT_3D('',#32240,#18314,#18315);
#14978=AXIS2_PLACEMENT_3D('',#32243,#18318,#18319);
#14979=AXIS2_PLACEMENT_3D('',#32244,#18320,#18321);
#14980=AXIS2_PLACEMENT_3D('',#32245,#18322,#18323);
#14981=AXIS2_PLACEMENT_3D('',#32248,#18326,#18327);
#14982=AXIS2_PLACEMENT_3D('',#32249,#18328,#18329);
#14983=AXIS2_PLACEMENT_3D('',#32250,#18330,#18331);
#14984=AXIS2_PLACEMENT_3D('',#32254,#18334,#18335);
#14985=AXIS2_PLACEMENT_3D('',#32258,#18338,#18339);
#14986=AXIS2_PLACEMENT_3D('',#32260,#18341,#18342);
#17904=DIRECTION('axis',(0.,0.,1.));
#17905=DIRECTION('refdir',(1.,0.,0.));
#17906=DIRECTION('center_axis',(-1.,0.,0.));
#17907=DIRECTION('ref_axis',(0.,0.,-1.));
#17908=DIRECTION('center_axis',(1.,0.,0.));
#17909=DIRECTION('ref_axis',(0.,0.,-1.));
#17910=DIRECTION('',(-0.707106781186548,-8.65956056235493E-17,0.707106781186547));
#17911=DIRECTION('center_axis',(-1.,0.,0.));
#17912=DIRECTION('ref_axis',(0.,0.,-1.));
#17913=DIRECTION('center_axis',(1.,0.,0.));
#17914=DIRECTION('ref_axis',(0.,0.,-1.));
#17915=DIRECTION('center_axis',(-1.,0.,0.));
#17916=DIRECTION('ref_axis',(0.,0.,-1.));
#17917=DIRECTION('',(-1.,0.,0.));
#17918=DIRECTION('center_axis',(1.,0.,0.));
#17919=DIRECTION('ref_axis',(0.,0.,-1.));
#17920=DIRECTION('',(0.,-0.309016994374948,0.951056516295153));
#17921=DIRECTION('',(0.,0.309016994374948,0.951056516295153));
#17922=DIRECTION('',(0.,0.809016994374947,0.587785252292473));
#17923=DIRECTION('',(0.,1.,-2.24547323617027E-16));
#17924=DIRECTION('',(0.,0.809016994374947,-0.587785252292473));
#17925=DIRECTION('',(0.,0.309016994374948,-0.951056516295153));
#17926=DIRECTION('',(0.,-0.309016994374948,-0.951056516295153));
#17927=DIRECTION('',(0.,-0.809016994374947,-0.587785252292473));
#17928=DIRECTION('',(0.,-1.,2.24547323617027E-16));
#17929=DIRECTION('',(0.,-0.809016994374947,0.587785252292473));
#17930=DIRECTION('center_axis',(1.,0.,0.));
#17931=DIRECTION('ref_axis',(0.,0.,-1.));
#17932=DIRECTION('center_axis',(1.,0.,0.));
#17933=DIRECTION('ref_axis',(0.,0.,-1.));
#17934=DIRECTION('',(-0.707106781186548,8.65956056235493E-17,-0.707106781186547));
#17935=DIRECTION('center_axis',(1.,0.,0.));
#17936=DIRECTION('ref_axis',(0.,0.,-1.));
#17937=DIRECTION('',(0.,0.951056516295154,0.309016994374947));
#17938=DIRECTION('',(0.,-0.309016994374948,0.951056516295154));
#17939=DIRECTION('',(0.,0.587785252292475,-0.809016994374946));
#17940=DIRECTION('',(0.,-0.809016994374947,0.587785252292473));
#17941=DIRECTION('',(0.,-0.587785252292473,-0.809016994374947));
#17942=DIRECTION('',(0.,0.809016994374947,-0.587785252292473));
#17943=DIRECTION('',(0.,0.587785252292473,0.809016994374947));
#17944=DIRECTION('',(0.,-0.809016994374947,0.587785252292473));
#17945=DIRECTION('',(0.,0.951056516295153,-0.30901699437495));
#17946=DIRECTION('',(0.,-1.,2.24547323617027E-16));
#17947=DIRECTION('',(0.,-5.55111512312578E-17,-1.));
#17948=DIRECTION('',(0.,1.,1.66533453693773E-16));
#17949=DIRECTION('',(0.,3.33066907387547E-16,1.));
#17950=DIRECTION('',(0.,-1.,2.24547323617027E-16));
#17951=DIRECTION('',(0.,0.951056516295154,0.309016994374946));
#17952=DIRECTION('',(0.,-0.809016994374947,-0.587785252292473));
#17953=DIRECTION('',(0.,0.587785252292473,-0.809016994374947));
#17954=DIRECTION('',(0.,0.809016994374947,0.587785252292473));
#17955=DIRECTION('',(0.,-0.587785252292473,0.809016994374948));
#17956=DIRECTION('',(0.,-0.809016994374947,-0.587785252292473));
#17957=DIRECTION('',(0.,0.587785252292478,0.809016994374944));
#17958=DIRECTION('',(0.,-0.309016994374948,-0.951056516295153));
#17959=DIRECTION('',(0.,0.951056516295153,-0.309016994374948));
#17960=DIRECTION('',(0.,0.309016994374947,0.951056516295154));
#17961=DIRECTION('',(0.,-0.951056516295153,0.309016994374948));
#17962=DIRECTION('',(0.,-0.309016994374948,-0.951056516295153));
#17963=DIRECTION('',(0.,0.,1.));
#17964=DIRECTION('',(0.,0.309016994374948,-0.951056516295153));
#17965=DIRECTION('',(0.,0.951056516295154,0.309016994374947));
#17966=DIRECTION('',(0.,-0.309016994374948,0.951056516295153));
#17967=DIRECTION('',(0.,-0.951056516295154,-0.309016994374947));
#17968=DIRECTION('',(0.,0.309016994374948,-0.951056516295154));
#17969=DIRECTION('',(0.,-0.587785252292475,0.809016994374946));
#17970=DIRECTION('',(0.,0.809016994374947,-0.587785252292473));
#17971=DIRECTION('',(0.,0.587785252292473,0.809016994374947));
#17972=DIRECTION('',(0.,-0.809016994374947,0.587785252292473));
#17973=DIRECTION('',(0.,-0.587785252292473,-0.809016994374947));
#17974=DIRECTION('',(0.,0.809016994374947,-0.587785252292473));
#17975=DIRECTION('',(0.,-0.951056516295154,0.309016994374947));
#17976=DIRECTION('',(0.,1.,-2.24547323617027E-16));
#17977=DIRECTION('',(0.,1.66533453693773E-16,1.));
#17978=DIRECTION('',(0.,-1.,-5.55111512312578E-17));
#17979=DIRECTION('',(0.,-4.44089209850063E-16,-1.));
#17980=DIRECTION('',(0.,1.,-2.24547323617027E-16));
#17981=DIRECTION('',(0.,-0.951056516295153,-0.309016994374949));
#17982=DIRECTION('',(0.,0.809016994374947,0.587785252292473));
#17983=DIRECTION('',(0.,-0.587785252292473,0.809016994374947));
#17984=DIRECTION('',(0.,-0.809016994374947,-0.587785252292473));
#17985=DIRECTION('',(0.,0.587785252292473,-0.809016994374948));
#17986=DIRECTION('',(0.,0.809016994374948,0.587785252292473));
#17987=DIRECTION('',(0.,-0.587785252292472,-0.809016994374948));
#17988=DIRECTION('',(0.,0.309016994374948,0.951056516295153));
#17989=DIRECTION('',(0.,-0.951056516295153,0.309016994374948));
#17990=DIRECTION('',(0.,-0.309016994374948,-0.951056516295154));
#17991=DIRECTION('',(0.,0.951056516295153,-0.309016994374948));
#17992=DIRECTION('',(0.,0.309016994374948,0.951056516295153));
#17993=DIRECTION('',(0.,0.,-1.));
#17994=DIRECTION('',(0.,-0.309016994374948,0.951056516295153));
#17995=DIRECTION('',(0.,-0.951056516295154,-0.309016994374947));
#17996=DIRECTION('',(0.,0.309016994374948,-0.951056516295153));
#17997=DIRECTION('center_axis',(0.707106781186548,0.672498511963957,0.218508012224411));
#17998=DIRECTION('ref_axis',(0.295241808844326,0.,-0.955422563220238));
#17999=DIRECTION('',(0.707106781186547,-0.672498511963958,-0.218508012224411));
#18000=DIRECTION('',(0.,-0.309016994374948,0.951056516295153));
#18001=DIRECTION('',(-0.707106781186547,0.672498511963958,0.218508012224411));
#18002=DIRECTION('center_axis',(0.,-0.951056516295154,-0.309016994374948));
#18003=DIRECTION('ref_axis',(0.,0.309016994374948,-0.951056516295153));
#18004=DIRECTION('',(1.,0.,0.));
#18005=DIRECTION('',(0.,-0.309016994374948,0.951056516295153));
#18006=DIRECTION('',(1.,0.,0.));
#18007=DIRECTION('center_axis',(0.707106781186547,0.415626937777453,0.572061402817685));
#18008=DIRECTION('ref_axis',(0.628960169645094,0.,-0.777437524821136));
#18009=DIRECTION('',(0.707106781186548,-0.415626937777453,-0.572061402817684));
#18010=DIRECTION('',(0.,-0.809016994374947,0.587785252292473));
#18011=DIRECTION('',(-0.707106781186548,0.415626937777453,0.572061402817684));
#18012=DIRECTION('center_axis',(0.,-0.587785252292473,-0.809016994374948));
#18013=DIRECTION('ref_axis',(0.,0.809016994374947,-0.587785252292473));
#18014=DIRECTION('',(1.,0.,0.));
#18015=DIRECTION('',(0.,-0.809016994374947,0.587785252292473));
#18016=DIRECTION('',(1.,0.,0.));
#18017=DIRECTION('center_axis',(0.707106781186548,-1.17756934401283E-16,
0.707106781186548));
#18018=DIRECTION('ref_axis',(0.707106781186548,0.,-0.707106781186548));
#18019=DIRECTION('',(0.707106781186548,-3.92523114670944E-17,-0.707106781186548));
#18020=DIRECTION('',(0.,-1.,-1.66533453693773E-16));
#18021=DIRECTION('',(-0.707106781186548,2.35513868802566E-16,0.707106781186548));
#18022=DIRECTION('center_axis',(0.,1.66533453693773E-16,-1.));
#18023=DIRECTION('ref_axis',(0.,1.,1.66533453693773E-16));
#18024=DIRECTION('',(1.,0.,0.));
#18025=DIRECTION('',(0.,-1.,-1.66533453693773E-16));
#18026=DIRECTION('',(1.,0.,0.));
#18027=DIRECTION('center_axis',(-0.596110861367214,0.649561473330963,0.471934034928767));
#18028=DIRECTION('ref_axis',(0.620713403652074,0.,0.784037544079783));
#18029=DIRECTION('',(0.,-0.587785252292475,0.809016994374946));
#18030=DIRECTION('',(0.638130334584325,0.740019202960846,-0.212511776926577));
#18031=DIRECTION('',(-0.638130334584329,-0.0265677996432243,-0.769469835734585));
#18032=DIRECTION('center_axis',(-0.707106781186548,0.672498511963956,0.21850801222441));
#18033=DIRECTION('ref_axis',(0.295241808844326,0.,0.955422563220239));
#18034=DIRECTION('',(-0.689151757774652,-0.724617040067447,-5.98775806539528E-15));
#18035=DIRECTION('',(0.,0.309016994374948,-0.951056516295153));
#18036=DIRECTION('',(-0.295241808844326,0.,-0.955422563220239));
#18037=DIRECTION('center_axis',(-0.596110861367212,0.248110405029972,0.763605308962624));
#18038=DIRECTION('ref_axis',(0.788252578093854,0.,0.615351828735718));
#18039=DIRECTION('',(0.,-0.951056516295153,0.30901699437495));
#18040=DIRECTION('',(0.638130334584327,0.723599399775037,0.263046734875194));
#18041=DIRECTION('',(-0.63813033458433,0.430789220114182,-0.638130334584327));
#18042=DIRECTION('center_axis',(-0.707106781186546,0.415626937777454,0.572061402817685));
#18043=DIRECTION('ref_axis',(0.628960169645095,0.,0.777437524821135));
#18044=DIRECTION('',(0.,0.809016994374947,-0.587785252292473));
#18045=DIRECTION('center_axis',(-0.596110861367212,-0.24811040502997,0.763605308962624));
#18046=DIRECTION('ref_axis',(0.788252578093855,0.,0.615351828735717));
#18047=DIRECTION('',(0.,-0.951056516295154,-0.309016994374946));
#18048=DIRECTION('',(0.638130334584328,0.430789220114187,0.638130334584326));
#18049=DIRECTION('',(-0.638130334584328,0.723599399775035,-0.263046734875197));
#18050=DIRECTION('center_axis',(-0.707106781186546,1.5877893522689E-16,
0.707106781186549));
#18051=DIRECTION('ref_axis',(0.707106781186549,0.,0.707106781186546));
#18052=DIRECTION('',(0.,1.,-2.24547323617027E-16));
#18053=DIRECTION('center_axis',(-0.707106781186546,-0.415626937777454,0.572061402817685));
#18054=DIRECTION('ref_axis',(0.628960169645095,0.,0.777437524821135));
#18055=DIRECTION('',(0.295241808844322,0.561583292368335,0.772953090454443));
#18056=DIRECTION('',(0.,0.809016994374947,0.587785252292473));
#18057=DIRECTION('',(0.689151757774653,-0.586227499828236,0.425919209711468));
#18058=DIRECTION('center_axis',(0.,-0.309016994374946,0.951056516295154));
#18059=DIRECTION('ref_axis',(1.,0.,0.));
#18060=DIRECTION('',(-1.,0.,0.));
#18061=DIRECTION('',(1.,0.,0.));
#18062=DIRECTION('center_axis',(0.,0.30901699437495,0.951056516295153));
#18063=DIRECTION('ref_axis',(1.,0.,0.));
#18064=DIRECTION('',(-1.,0.,0.));
#18065=DIRECTION('',(1.,0.,0.));
#18066=DIRECTION('center_axis',(0.,0.809016994374946,0.587785252292475));
#18067=DIRECTION('ref_axis',(1.,0.,0.));
#18068=DIRECTION('',(-1.,0.,0.));
#18069=DIRECTION('',(1.,0.,0.));
#18070=DIRECTION('center_axis',(0.,0.587785252292473,0.809016994374947));
#18071=DIRECTION('ref_axis',(0.,-0.809016994374947,0.587785252292473));
#18072=DIRECTION('',(-1.,0.,0.));
#18073=DIRECTION('',(0.,0.809016994374947,-0.587785252292473));
#18074=DIRECTION('',(1.,0.,0.));
#18075=DIRECTION('center_axis',(0.,2.24547323617027E-16,1.));
#18076=DIRECTION('ref_axis',(0.,-1.,2.24547323617027E-16));
#18077=DIRECTION('',(-1.,0.,0.));
#18078=DIRECTION('',(0.,1.,-2.24547323617027E-16));
#18079=DIRECTION('',(1.,0.,0.));
#18080=DIRECTION('center_axis',(0.,-0.587785252292473,0.809016994374947));
#18081=DIRECTION('ref_axis',(0.,-0.809016994374947,-0.587785252292473));
#18082=DIRECTION('',(-1.,0.,0.));
#18083=DIRECTION('',(-1.,0.,0.));
#18084=DIRECTION('',(0.,0.809016994374947,0.587785252292473));
#18085=DIRECTION('',(1.,0.,0.));
#18086=DIRECTION('center_axis',(0.,-0.809016994374944,0.587785252292478));
#18087=DIRECTION('ref_axis',(1.,0.,0.));
#18088=DIRECTION('',(-0.295241808844332,0.561583292368333,0.77295309045444));
#18089=DIRECTION('',(1.,0.,0.));
#18090=DIRECTION('center_axis',(-0.707106781186547,-0.672498511963958,0.218508012224411));
#18091=DIRECTION('ref_axis',(0.295241808844327,0.,0.955422563220238));
#18092=DIRECTION('',(0.638130334584329,-0.473776822943218,0.60689801295203));
#18093=DIRECTION('',(0.,0.309016994374948,0.951056516295153));
#18094=DIRECTION('center_axis',(0.707106781186548,-0.415626937777453,0.572061402817684));
#18095=DIRECTION('ref_axis',(0.628960169645094,0.,-0.777437524821136));
#18096=DIRECTION('',(0.707106781186547,0.415626937777454,-0.572061402817685));
#18097=DIRECTION('',(0.,-0.809016994374947,-0.587785252292473));
#18098=DIRECTION('',(-0.707106781186547,-0.415626937777453,0.572061402817685));
#18099=DIRECTION('center_axis',(0.,0.587785252292473,-0.809016994374947));
#18100=DIRECTION('ref_axis',(0.,0.809016994374947,0.587785252292473));
#18101=DIRECTION('',(1.,0.,0.));
#18102=DIRECTION('',(0.,-0.809016994374947,-0.587785252292473));
#18103=DIRECTION('',(1.,0.,0.));
#18104=DIRECTION('center_axis',(0.707106781186546,-0.672498511963958,0.218508012224411));
#18105=DIRECTION('ref_axis',(0.295241808844327,0.,-0.955422563220238));
#18106=DIRECTION('',(0.707106781186549,0.672498511963956,-0.21850801222441));
#18107=DIRECTION('',(0.,-0.309016994374947,-0.951056516295154));
#18108=DIRECTION('',(-0.707106781186549,-0.672498511963956,0.21850801222441));
#18109=DIRECTION('center_axis',(0.,0.951056516295154,-0.309016994374947));
#18110=DIRECTION('ref_axis',(0.,0.309016994374947,0.951056516295154));
#18111=DIRECTION('',(1.,0.,0.));
#18112=DIRECTION('',(0.,-0.309016994374947,-0.951056516295154));
#18113=DIRECTION('',(1.,0.,0.));
#18114=DIRECTION('center_axis',(0.707106781186546,-0.672498511963958,-0.218508012224411));
#18115=DIRECTION('ref_axis',(-0.295241808844327,0.,-0.955422563220238));
#18116=DIRECTION('',(0.707106781186549,0.672498511963956,0.21850801222441));
#18117=DIRECTION('',(0.,0.309016994374948,-0.951056516295153));
#18118=DIRECTION('',(-0.707106781186549,-0.672498511963956,-0.21850801222441));
#18119=DIRECTION('center_axis',(0.,0.951056516295154,0.309016994374948));
#18120=DIRECTION('ref_axis',(0.,-0.309016994374948,0.951056516295153));
#18121=DIRECTION('',(1.,0.,0.));
#18122=DIRECTION('',(0.,0.309016994374948,-0.951056516295153));
#18123=DIRECTION('',(1.,0.,0.));
#18124=DIRECTION('center_axis',(0.707106781186545,-0.415626937777455,-0.572061402817686));
#18125=DIRECTION('ref_axis',(-0.628960169645096,0.,-0.777437524821134));
#18126=DIRECTION('',(0.70710678118655,0.415626937777452,0.572061402817683));
#18127=DIRECTION('',(0.,0.809016994374947,-0.587785252292473));
#18128=DIRECTION('',(-0.70710678118655,-0.415626937777452,-0.572061402817682));
#18129=DIRECTION('center_axis',(0.,0.587785252292473,0.809016994374948));
#18130=DIRECTION('ref_axis',(0.,-0.809016994374947,0.587785252292473));
#18131=DIRECTION('',(1.,0.,0.));
#18132=DIRECTION('',(0.,0.809016994374947,-0.587785252292473));
#18133=DIRECTION('',(1.,0.,0.));
#18134=DIRECTION('center_axis',(0.707106781186548,3.92523114670944E-17,
-0.707106781186548));
#18135=DIRECTION('ref_axis',(-0.707106781186548,0.,-0.707106781186548));
#18136=DIRECTION('',(0.707106781186548,1.17756934401283E-16,0.707106781186548));
#18137=DIRECTION('',(0.,1.,5.55111512312578E-17));
#18138=DIRECTION('',(-0.707106781186548,-3.14018491736755E-16,-0.707106781186548));
#18139=DIRECTION('center_axis',(0.,-5.55111512312578E-17,1.));
#18140=DIRECTION('ref_axis',(0.,-1.,-5.55111512312578E-17));
#18141=DIRECTION('',(1.,0.,0.));
#18142=DIRECTION('',(0.,1.,5.55111512312578E-17));
#18143=DIRECTION('',(1.,0.,0.));
#18144=DIRECTION('center_axis',(0.707106781186548,0.415626937777453,-0.572061402817684));
#18145=DIRECTION('ref_axis',(-0.628960169645094,0.,-0.777437524821136));
#18146=DIRECTION('',(0.707106781186547,-0.415626937777454,0.572061402817685));
#18147=DIRECTION('',(0.,0.809016994374947,0.587785252292473));
#18148=DIRECTION('',(-0.707106781186547,0.415626937777453,-0.572061402817685));
#18149=DIRECTION('center_axis',(0.,-0.587785252292473,0.809016994374947));
#18150=DIRECTION('ref_axis',(0.,-0.809016994374947,-0.587785252292473));
#18151=DIRECTION('',(1.,0.,0.));
#18152=DIRECTION('',(0.,0.809016994374947,0.587785252292473));
#18153=DIRECTION('',(1.,0.,0.));
#18154=DIRECTION('center_axis',(-0.596110861367213,-0.80290213660199,0.));
#18155=DIRECTION('ref_axis',(0.,0.,1.));
#18156=DIRECTION('',(0.,0.,-1.));
#18157=DIRECTION('',(-0.638130334584328,0.473776822943217,0.606898012952033));
#18158=DIRECTION('center_axis',(-0.596110861367212,-0.649561473330965,-0.471934034928767));
#18159=DIRECTION('ref_axis',(-0.620713403652076,0.,0.784037544079782));
#18160=DIRECTION('',(0.,0.587785252292475,-0.809016994374946));
#18161=DIRECTION('',(0.638130334584328,-0.740019202960844,0.212511776926575));
#18162=DIRECTION('',(-0.638130334584327,0.0265677996432183,0.769469835734587));
#18163=DIRECTION('center_axis',(-0.707106781186547,-0.672498511963958,-0.218508012224411));
#18164=DIRECTION('ref_axis',(-0.295241808844327,0.,0.955422563220238));
#18165=DIRECTION('',(0.,-0.309016994374948,0.951056516295153));
#18166=DIRECTION('center_axis',(-0.596110861367213,-0.248110405029968,-0.763605308962624));
#18167=DIRECTION('ref_axis',(-0.788252578093854,0.,0.615351828735718));
#18168=DIRECTION('',(0.,0.951056516295154,-0.309016994374947));
#18169=DIRECTION('',(0.638130334584328,-0.723599399775034,-0.2630467348752));
#18170=DIRECTION('',(-0.638130334584328,-0.430789220114189,0.638130334584325));
#18171=DIRECTION('center_axis',(-0.707106781186546,-0.415626937777454,-0.572061402817685));
#18172=DIRECTION('ref_axis',(-0.628960169645095,0.,0.777437524821135));
#18173=DIRECTION('',(0.,-0.809016994374947,0.587785252292473));
#18174=DIRECTION('center_axis',(-0.596110861367212,0.248110405029972,-0.763605308962624));
#18175=DIRECTION('ref_axis',(-0.788252578093855,0.,0.615351828735717));
#18176=DIRECTION('',(0.,0.951056516295153,0.309016994374949));
#18177=DIRECTION('',(0.638130334584329,-0.430789220114185,-0.638130334584327));
#18178=DIRECTION('',(-0.638130334584327,-0.723599399775037,0.263046734875194));
#18179=DIRECTION('center_axis',(-0.707106781186546,-1.5877893522689E-16,
-0.707106781186549));
#18180=DIRECTION('ref_axis',(-0.707106781186549,0.,0.707106781186546));
#18181=DIRECTION('',(0.,-1.,2.24547323617027E-16));
#18182=DIRECTION('center_axis',(-0.596110861367213,0.649561473330965,-0.471934034928765));
#18183=DIRECTION('ref_axis',(-0.620713403652073,0.,0.784037544079784));
#18184=DIRECTION('',(0.638130334584328,0.0265677996432242,-0.769469835734586));
#18185=DIRECTION('',(-0.638130334584328,-0.740019202960844,-0.212511776926575));
#18186=DIRECTION('',(0.,0.587785252292472,0.809016994374948));
#18187=DIRECTION('center_axis',(-0.707106781186547,0.672498511963958,-0.218508012224411));
#18188=DIRECTION('ref_axis',(-0.295241808844327,0.,0.955422563220238));
#18189=DIRECTION('',(0.295241808844329,0.,-0.955422563220238));
#18190=DIRECTION('',(0.,-0.309016994374948,-0.951056516295153));
#18191=DIRECTION('center_axis',(0.,0.809016994374948,-0.587785252292472));
#18192=DIRECTION('ref_axis',(-1.,0.,0.));
#18193=DIRECTION('',(-1.,0.,0.));
#18194=DIRECTION('',(1.,0.,0.));
#18195=DIRECTION('center_axis',(-0.707106781186546,0.415626937777454,-0.572061402817685));
#18196=DIRECTION('ref_axis',(-0.628960169645095,0.,0.777437524821135));
#18197=DIRECTION('',(0.,-0.809016994374947,-0.587785252292473));
#18198=DIRECTION('center_axis',(0.,1.,0.));
#18199=DIRECTION('ref_axis',(0.,0.,1.));
#18200=DIRECTION('',(1.,0.,0.));
#18201=DIRECTION('',(-1.,0.,0.));
#18202=DIRECTION('center_axis',(0.,0.309016994374949,-0.951056516295153));
#18203=DIRECTION('ref_axis',(-1.,0.,0.));
#18204=DIRECTION('',(-1.,0.,0.));
#18205=DIRECTION('',(1.,0.,0.));
#18206=DIRECTION('center_axis',(0.,-0.309016994374947,-0.951056516295154));
#18207=DIRECTION('ref_axis',(-1.,0.,0.));
#18208=DIRECTION('',(-1.,0.,0.));
#18209=DIRECTION('',(1.,0.,0.));
#18210=DIRECTION('center_axis',(0.,-0.809016994374946,-0.587785252292475));
#18211=DIRECTION('ref_axis',(-1.,0.,0.));
#18212=DIRECTION('',(-1.,0.,0.));
#18213=DIRECTION('',(1.,0.,0.));
#18214=DIRECTION('center_axis',(0.,-1.,0.));
#18215=DIRECTION('ref_axis',(0.,0.,-1.));
#18216=DIRECTION('',(-1.,0.,0.));
#18217=DIRECTION('',(1.,0.,0.));
#18218=DIRECTION('center_axis',(0.,-0.951056516295154,0.309016994374948));
#18219=DIRECTION('ref_axis',(0.,-0.309016994374948,-0.951056516295153));
#18220=DIRECTION('',(-1.,0.,0.));
#18221=DIRECTION('',(0.,0.309016994374948,0.951056516295153));
#18222=DIRECTION('',(1.,0.,0.));
#18223=DIRECTION('center_axis',(0.,-0.951056516295154,-0.309016994374948));
#18224=DIRECTION('ref_axis',(0.,0.309016994374948,-0.951056516295153));
#18225=DIRECTION('',(-1.,0.,0.));
#18226=DIRECTION('',(0.,-0.309016994374948,0.951056516295153));
#18227=DIRECTION('',(1.,0.,0.));
#18228=DIRECTION('center_axis',(0.,-0.587785252292473,-0.809016994374947));
#18229=DIRECTION('ref_axis',(0.,0.809016994374947,-0.587785252292473));
#18230=DIRECTION('',(-1.,0.,0.));
#18231=DIRECTION('',(0.,-0.809016994374947,0.587785252292473));
#18232=DIRECTION('',(1.,0.,0.));
#18233=DIRECTION('center_axis',(0.,-2.24547323617027E-16,-1.));
#18234=DIRECTION('ref_axis',(0.,1.,-2.24547323617027E-16));
#18235=DIRECTION('',(-1.,0.,0.));
#18236=DIRECTION('',(0.,-1.,2.24547323617027E-16));
#18237=DIRECTION('',(1.,0.,0.));
#18238=DIRECTION('center_axis',(0.,0.587785252292473,-0.809016994374948));
#18239=DIRECTION('ref_axis',(0.,0.809016994374947,0.587785252292473));
#18240=DIRECTION('',(-1.,0.,0.));
#18241=DIRECTION('',(0.,-0.809016994374947,-0.587785252292473));
#18242=DIRECTION('',(1.,0.,0.));
#18243=DIRECTION('center_axis',(0.707106781186546,0.672498511963958,-0.218508012224411));
#18244=DIRECTION('ref_axis',(-0.295241808844327,0.,-0.955422563220238));
#18245=DIRECTION('',(0.707106781186549,-0.672498511963956,0.21850801222441));
#18246=DIRECTION('',(0.,0.309016994374948,0.951056516295154));
#18247=DIRECTION('',(-0.707106781186549,0.672498511963956,-0.218508012224411));
#18248=DIRECTION('center_axis',(0.,-0.951056516295154,0.309016994374948));
#18249=DIRECTION('ref_axis',(0.,-0.309016994374948,-0.951056516295154));
#18250=DIRECTION('',(1.,0.,0.));
#18251=DIRECTION('',(0.,0.309016994374948,0.951056516295154));
#18252=DIRECTION('',(1.,0.,0.));
#18253=DIRECTION('center_axis',(1.,0.,0.));
#18254=DIRECTION('ref_axis',(0.,-0.587785252292473,-0.809016994374947));
#18255=DIRECTION('',(0.,-0.309016994374948,-0.951056516295153));
#18256=DIRECTION('',(0.,0.951056516295153,-0.309016994374948));
#18257=DIRECTION('',(0.,-0.951056516295153,0.309016994374948));
#18258=DIRECTION('center_axis',(0.,-0.309016994374948,-0.951056516295154));
#18259=DIRECTION('ref_axis',(0.,0.951056516295153,-0.309016994374948));
#18260=DIRECTION('',(1.,0.,0.));
#18261=DIRECTION('center_axis',(0.,0.309016994374948,0.951056516295153));
#18262=DIRECTION('ref_axis',(0.,-0.951056516295153,0.309016994374948));
#18263=DIRECTION('',(-1.,0.,0.));
#18264=DIRECTION('center_axis',(0.,0.951056516295154,-0.309016994374948));
#18265=DIRECTION('ref_axis',(0.,0.309016994374948,0.951056516295153));
#18266=DIRECTION('center_axis',(1.,0.,0.));
#18267=DIRECTION('ref_axis',(0.,-0.951056516295154,-0.309016994374947));
#18268=DIRECTION('',(0.,0.587785252292473,-0.809016994374948));
#18269=DIRECTION('',(0.,-0.587785252292473,0.809016994374947));
#18270=DIRECTION('center_axis',(0.,-0.809016994374948,-0.587785252292473));
#18271=DIRECTION('ref_axis',(0.,0.587785252292473,-0.809016994374947));
#18272=DIRECTION('center_axis',(0.,0.809016994374948,0.587785252292473));
#18273=DIRECTION('ref_axis',(0.,-0.587785252292473,0.809016994374948));
#18274=DIRECTION('center_axis',(1.,0.,0.));
#18275=DIRECTION('ref_axis',(0.,-0.951056516295153,0.309016994374948));
#18276=DIRECTION('',(0.,-4.44089209850063E-16,-1.));
#18277=DIRECTION('',(0.,1.66533453693773E-16,1.));
#18278=DIRECTION('center_axis',(0.,-1.,1.66533453693773E-16));
#18279=DIRECTION('ref_axis',(0.,-1.66533453693773E-16,-1.));
#18280=DIRECTION('center_axis',(0.,1.,-4.44089209850063E-16));
#18281=DIRECTION('ref_axis',(0.,4.44089209850063E-16,1.));
#18282=DIRECTION('center_axis',(1.,0.,0.));
#18283=DIRECTION('ref_axis',(0.,-0.587785252292473,0.809016994374947));
#18284=DIRECTION('',(0.,-0.587785252292473,-0.809016994374947));
#18285=DIRECTION('',(0.,0.587785252292473,0.809016994374947));
#18286=DIRECTION('center_axis',(0.,-0.809016994374947,0.587785252292473));
#18287=DIRECTION('ref_axis',(0.,-0.587785252292473,-0.809016994374947));
#18288=DIRECTION('center_axis',(0.,0.809016994374947,-0.587785252292473));
#18289=DIRECTION('ref_axis',(0.,0.587785252292473,0.809016994374947));
#18290=DIRECTION('center_axis',(1.,0.,0.));
#18291=DIRECTION('ref_axis',(0.,1.22464679914735E-16,1.));
#18292=DIRECTION('',(0.,-0.951056516295154,-0.309016994374947));
#18293=DIRECTION('',(0.,0.951056516295154,0.309016994374947));
#18294=DIRECTION('center_axis',(0.,-0.309016994374947,0.951056516295154));
#18295=DIRECTION('ref_axis',(0.,-0.951056516295154,-0.309016994374947));
#18296=DIRECTION('center_axis',(0.,0.309016994374947,-0.951056516295154));
#18297=DIRECTION('ref_axis',(0.,0.951056516295154,0.309016994374947));
#18298=DIRECTION('center_axis',(1.,0.,0.));
#18299=DIRECTION('ref_axis',(0.,0.587785252292473,0.809016994374947));
#18300=DIRECTION('',(0.,-0.951056516295153,0.309016994374948));
#18301=DIRECTION('',(0.,0.951056516295153,-0.309016994374948));
#18302=DIRECTION('center_axis',(0.,0.309016994374948,0.951056516295154));
#18303=DIRECTION('ref_axis',(0.,-0.951056516295153,0.309016994374948));
#18304=DIRECTION('center_axis',(0.,-0.309016994374948,-0.951056516295154));
#18305=DIRECTION('ref_axis',(0.,0.951056516295153,-0.309016994374948));
#18306=DIRECTION('center_axis',(1.,0.,0.));
#18307=DIRECTION('ref_axis',(0.,0.951056516295154,0.309016994374947));
#18308=DIRECTION('',(0.,-0.587785252292473,0.809016994374948));
#18309=DIRECTION('',(0.,0.587785252292473,-0.809016994374947));
#18310=DIRECTION('center_axis',(0.,0.809016994374948,0.587785252292473));
#18311=DIRECTION('ref_axis',(0.,-0.587785252292473,0.809016994374947));
#18312=DIRECTION('center_axis',(0.,-0.809016994374948,-0.587785252292473));
#18313=DIRECTION('ref_axis',(0.,0.587785252292473,-0.809016994374948));
#18314=DIRECTION('center_axis',(1.,0.,0.));
#18315=DIRECTION('ref_axis',(0.,0.951056516295154,-0.309016994374948));
#18316=DIRECTION('',(0.,3.33066907387547E-16,1.));
#18317=DIRECTION('',(0.,-5.55111512312578E-17,-1.));
#18318=DIRECTION('center_axis',(0.,1.,-5.55111512312578E-17));
#18319=DIRECTION('ref_axis',(0.,5.55111512312578E-17,1.));
#18320=DIRECTION('center_axis',(0.,-1.,3.33066907387547E-16));
#18321=DIRECTION('ref_axis',(0.,-3.33066907387547E-16,-1.));
#18322=DIRECTION('center_axis',(1.,0.,0.));
#18323=DIRECTION('ref_axis',(0.,0.587785252292473,-0.809016994374947));
#18324=DIRECTION('',(0.,0.587785252292473,0.809016994374947));
#18325=DIRECTION('',(0.,-0.587785252292473,-0.809016994374947));
#18326=DIRECTION('center_axis',(0.,0.809016994374947,-0.587785252292473));
#18327=DIRECTION('ref_axis',(0.,0.587785252292473,0.809016994374947));
#18328=DIRECTION('center_axis',(0.,-0.809016994374947,0.587785252292473));
#18329=DIRECTION('ref_axis',(0.,-0.587785252292473,-0.809016994374947));
#18330=DIRECTION('center_axis',(0.,0.309016994374947,-0.951056516295154));
#18331=DIRECTION('ref_axis',(0.,0.951056516295154,0.309016994374947));
#18332=DIRECTION('',(1.,0.,0.));
#18333=DIRECTION('',(0.,-0.951056516295154,-0.309016994374947));
#18334=DIRECTION('center_axis',(0.,-0.309016994374947,0.951056516295154));
#18335=DIRECTION('ref_axis',(0.,-0.951056516295154,-0.309016994374947));
#18336=DIRECTION('',(-1.,0.,0.));
#18337=DIRECTION('',(0.,0.951056516295154,0.309016994374947));
#18338=DIRECTION('center_axis',(1.,0.,0.));
#18339=DIRECTION('ref_axis',(0.,0.,-1.));
#18340=DIRECTION('',(0.,0.309016994374948,-0.951056516295153));
#18341=DIRECTION('center_axis',(0.,0.951056516295154,0.309016994374948));
#18342=DIRECTION('ref_axis',(0.,-0.309016994374948,0.951056516295153));
#31764=CARTESIAN_POINT('',(0.,0.,0.));
#31765=CARTESIAN_POINT('Origin',(0.12,0.,0.));
#31766=CARTESIAN_POINT('',(0.24,-1.95943487863577E-16,1.6));
#31767=CARTESIAN_POINT('Origin',(0.24,0.,0.));
#31768=CARTESIAN_POINT('',(0.,2.25335011043113E-16,1.84));
#31769=CARTESIAN_POINT('',(0.12,-2.10639249453345E-16,1.72));
#31770=CARTESIAN_POINT('Origin',(0.,0.,0.));
#31771=CARTESIAN_POINT('Origin',(0.,0.,0.));
#31772=CARTESIAN_POINT('',(5.76,1.95943487863577E-16,1.6));
#31773=CARTESIAN_POINT('Origin',(5.76,0.,0.));
#31774=CARTESIAN_POINT('',(0.,-1.95943487863577E-16,1.6));
#31775=CARTESIAN_POINT('Origin',(0.,0.,0.));
#31776=CARTESIAN_POINT('',(0.,7.74764906618282,-2.22044604925031E-15));
#31777=CARTESIAN_POINT('',(0.,6.26797976099509,4.55395386103981));
#31778=CARTESIAN_POINT('',(0.,7.38978042483906,1.10140642593496));
#31779=CARTESIAN_POINT('',(0.,6.26797976099509,-4.55395386103981));
#31780=CARTESIAN_POINT('',(0.,6.62584840233885,-3.45254743510485));
#31781=CARTESIAN_POINT('',(0.,2.39415522790368,-7.36845213036123));
#31782=CARTESIAN_POINT('',(0.,3.33106749444938,-6.68774552370588));
#31783=CARTESIAN_POINT('',(0.,-2.39415522790368,-7.36845213036123));
#31784=CARTESIAN_POINT('',(0.,-1.23606797749979,-7.36845213036123));
#31785=CARTESIAN_POINT('',(0.,-6.26797976099509,-4.55395386103981));
#31786=CARTESIAN_POINT('',(0.,-5.33106749444939,-5.23466046769516));
#31787=CARTESIAN_POINT('',(0.,-7.74764906618282,1.38777878078145E-15));
#31788=CARTESIAN_POINT('',(0.,-7.38978042483906,-1.10140642593496));
#31789=CARTESIAN_POINT('',(0.,-6.26797976099509,4.55395386103981));
#31790=CARTESIAN_POINT('',(0.,-6.62584840233885,3.45254743510485));
#31791=CARTESIAN_POINT('',(0.,-2.39415522790368,7.36845213036123));
#31792=CARTESIAN_POINT('',(0.,-3.33106749444939,6.68774552370588));
#31793=CARTESIAN_POINT('',(0.,2.39415522790368,7.36845213036123));
#31794=CARTESIAN_POINT('',(0.,1.23606797749979,7.36845213036123));
#31795=CARTESIAN_POINT('',(0.,5.33106749444939,5.23466046769516));
#31796=CARTESIAN_POINT('Origin',(5.88,0.,0.));
#31797=CARTESIAN_POINT('',(6.,-2.25335011043113E-16,1.84));
#31798=CARTESIAN_POINT('Origin',(6.,0.,0.));
#31799=CARTESIAN_POINT('',(5.88,-2.10639249453345E-16,1.72));
#31800=CARTESIAN_POINT('Origin',(6.,0.,0.));
#31801=CARTESIAN_POINT('',(6.,6.25657141382095,3.29463795232411));
#31802=CARTESIAN_POINT('',(6.,6.86524758424985,3.49240882872408));
#31803=CARTESIAN_POINT('',(6.,3.5325305503885,2.40954342245162));
#31804=CARTESIAN_POINT('',(6.,6.54630003364957,4.47402845442895));
#31805=CARTESIAN_POINT('',(6.,8.,0.));
#31806=CARTESIAN_POINT('',(6.,6.27797187634959,4.84335047888998));
#31807=CARTESIAN_POINT('',(6.,6.41213595499957,4.65868946665947));
#31808=CARTESIAN_POINT('',(6.,5.44295634824952,5.45002477159954));
#31809=CARTESIAN_POINT('',(6.,6.47213595499958,4.70228201833979));
#31810=CARTESIAN_POINT('',(6.,5.06677378678233,4.93225389519957));
#31811=CARTESIAN_POINT('',(6.,3.08933132029123,2.2105378355493));
#31812=CARTESIAN_POINT('',(6.,3.12513300028246,6.34293850070151));
#31813=CARTESIAN_POINT('',(6.,3.61054319690743,5.99026734932602));
#31814=CARTESIAN_POINT('',(6.,3.50131556174964,6.86070937710148));
#31815=CARTESIAN_POINT('',(6.,1.44158315993759,4.02573093823871));
#31816=CARTESIAN_POINT('',(6.,2.66630003364957,7.46738366981103));
#31817=CARTESIAN_POINT('',(6.,6.47213595499958,4.70228201833979));
#31818=CARTESIAN_POINT('',(6.,2.23213595499958,7.60845213036123));
#31819=CARTESIAN_POINT('',(6.,2.44921799432458,7.53791790008613));
#31820=CARTESIAN_POINT('',(6.,1.2,7.60845213036123));
#31821=CARTESIAN_POINT('',(6.,2.47213595499958,7.60845213036123));
#31822=CARTESIAN_POINT('',(6.,1.2,6.96845213036123));
#31823=CARTESIAN_POINT('',(6.,1.2,3.60422606518061));
#31824=CARTESIAN_POINT('',(6.,-1.2,6.96845213036123));
#31825=CARTESIAN_POINT('',(6.,-0.6,6.96845213036123));
#31826=CARTESIAN_POINT('',(6.,-1.2,7.60845213036123));
#31827=CARTESIAN_POINT('',(6.,-1.2,4.10422606518061));
#31828=CARTESIAN_POINT('',(6.,-2.23213595499958,7.60845213036123));
#31829=CARTESIAN_POINT('',(6.,2.47213595499958,7.60845213036123));
#31830=CARTESIAN_POINT('',(6.,-2.66630003364957,7.46738366981104));
#31831=CARTESIAN_POINT('',(6.,-2.44921799432457,7.53791790008613));
#31832=CARTESIAN_POINT('',(6.,-3.50131556174964,6.86070937710148));
#31833=CARTESIAN_POINT('',(6.,-2.47213595499958,7.60845213036123));
#31834=CARTESIAN_POINT('',(6.,-3.12513300028246,6.34293850070151));
#31835=CARTESIAN_POINT('',(6.,-1.14769053379136,3.62122244105123));
#31836=CARTESIAN_POINT('',(6.,-5.06677378678233,4.93225389519957));
#31837=CARTESIAN_POINT('',(6.,-4.58136359015736,5.28492504657506));
#31838=CARTESIAN_POINT('',(6.,-5.44295634824952,5.45002477159954));
#31839=CARTESIAN_POINT('',(6.,-3.38322394643747,2.61504633273677));
#31840=CARTESIAN_POINT('',(6.,-6.27797187634959,4.84335047888998));
#31841=CARTESIAN_POINT('',(6.,-2.47213595499958,7.60845213036123));
#31842=CARTESIAN_POINT('',(6.,-6.54630003364956,4.47402845442895));
#31843=CARTESIAN_POINT('',(6.,-6.41213595499956,4.65868946665949));
#31844=CARTESIAN_POINT('',(6.,-6.86524758424985,3.49240882872408));
#31845=CARTESIAN_POINT('',(6.,-6.47213595499958,4.70228201833979));
#31846=CARTESIAN_POINT('',(6.,-6.25657141382095,3.29463795232411));
#31847=CARTESIAN_POINT('',(6.,-3.05700229224093,2.25503492526414));
#31848=CARTESIAN_POINT('',(6.,-6.99821220032083,1.01210231321574));
#31849=CARTESIAN_POINT('',(6.,-6.81280200369586,1.58273622299283));
#31850=CARTESIAN_POINT('',(6.,-7.60688837074973,1.20987318961571));
#31851=CARTESIAN_POINT('',(6.,-4.27417133688838,0.127007783343246));
#31852=CARTESIAN_POINT('',(6.,-7.92583592135001,0.228253563910838));
#31853=CARTESIAN_POINT('',(6.,-6.47213595499958,4.70228201833979));
#31854=CARTESIAN_POINT('',(6.,-7.92583592135001,-0.228253563910836));
#31855=CARTESIAN_POINT('',(6.,-7.92583592135001,4.68375338513738E-16));
#31856=CARTESIAN_POINT('',(6.,-7.60688837074973,-1.20987318961571));
#31857=CARTESIAN_POINT('',(6.,-8.,9.79717439317883E-16));
#31858=CARTESIAN_POINT('',(6.,-6.99821220032083,-1.01210231321574));
#31859=CARTESIAN_POINT('',(6.,-3.7986430787408,0.0275007138442283));
#31860=CARTESIAN_POINT('',(6.,-6.25657141382095,-3.29463795232411));
#31861=CARTESIAN_POINT('',(6.,-6.44198161044592,-2.72400404254702));
#31862=CARTESIAN_POINT('',(6.,-6.86524758424985,-3.49240882872408));
#31863=CARTESIAN_POINT('',(6.,-3.5325305503885,-2.40954342245161));
#31864=CARTESIAN_POINT('',(6.,-6.54630003364957,-4.47402845442895));
#31865=CARTESIAN_POINT('',(6.,-8.,9.79717439317883E-16));
#31866=CARTESIAN_POINT('',(6.,-6.27797187634959,-4.84335047888998));
#31867=CARTESIAN_POINT('',(6.,-6.41213595499957,-4.65868946665947));
#31868=CARTESIAN_POINT('',(6.,-5.44295634824952,-5.45002477159954));
#31869=CARTESIAN_POINT('',(6.,-6.47213595499958,-4.70228201833978));
#31870=CARTESIAN_POINT('',(6.,-5.06677378678233,-4.93225389519957));
#31871=CARTESIAN_POINT('',(6.,-3.08933132029123,-2.2105378355493));
#31872=CARTESIAN_POINT('',(6.,-3.12513300028246,-6.34293850070151));
#31873=CARTESIAN_POINT('',(6.,-3.61054319690743,-5.99026734932603));
#31874=CARTESIAN_POINT('',(6.,-3.50131556174964,-6.86070937710148));
#31875=CARTESIAN_POINT('',(6.,-1.44158315993759,-4.02573093823871));
#31876=CARTESIAN_POINT('',(6.,-2.66630003364957,-7.46738366981103));
#31877=CARTESIAN_POINT('',(6.,-6.47213595499958,-4.70228201833978));
#31878=CARTESIAN_POINT('',(6.,-2.23213595499958,-7.60845213036123));
#31879=CARTESIAN_POINT('',(6.,-2.44921799432457,-7.53791790008613));
#31880=CARTESIAN_POINT('',(6.,-1.2,-7.60845213036123));
#31881=CARTESIAN_POINT('',(6.,-2.47213595499958,-7.60845213036123));
#31882=CARTESIAN_POINT('',(6.,-1.2,-6.96845213036123));
#31883=CARTESIAN_POINT('',(6.,-1.2,-3.60422606518061));
#31884=CARTESIAN_POINT('',(6.,1.2,-6.96845213036123));
#31885=CARTESIAN_POINT('',(6.,0.6,-6.96845213036123));
#31886=CARTESIAN_POINT('',(6.,1.2,-7.60845213036123));
#31887=CARTESIAN_POINT('',(6.,1.2,-4.10422606518061));
#31888=CARTESIAN_POINT('',(6.,2.23213595499958,-7.60845213036123));
#31889=CARTESIAN_POINT('',(6.,-2.47213595499958,-7.60845213036123));
#31890=CARTESIAN_POINT('',(6.,2.66630003364957,-7.46738366981103));
#31891=CARTESIAN_POINT('',(6.,2.44921799432458,-7.53791790008613));
#31892=CARTESIAN_POINT('',(6.,3.50131556174964,-6.86070937710148));
#31893=CARTESIAN_POINT('',(6.,2.47213595499958,-7.60845213036123));
#31894=CARTESIAN_POINT('',(6.,3.12513300028246,-6.34293850070151));
#31895=CARTESIAN_POINT('',(6.,1.14769053379136,-3.62122244105123));
#31896=CARTESIAN_POINT('',(6.,5.06677378678233,-4.93225389519957));
#31897=CARTESIAN_POINT('',(6.,4.58136359015736,-5.28492504657506));
#31898=CARTESIAN_POINT('',(6.,5.44295634824952,-5.45002477159954));
#31899=CARTESIAN_POINT('',(6.,3.38322394643747,-2.61504633273677));
#31900=CARTESIAN_POINT('',(6.,6.27797187634959,-4.84335047888998));
#31901=CARTESIAN_POINT('',(6.,2.47213595499958,-7.60845213036123));
#31902=CARTESIAN_POINT('',(6.,6.54630003364957,-4.47402845442895));
#31903=CARTESIAN_POINT('',(6.,6.41213595499958,-4.65868946665946));
#31904=CARTESIAN_POINT('',(6.,6.86524758424985,-3.49240882872408));
#31905=CARTESIAN_POINT('',(6.,6.47213595499958,-4.70228201833979));
#31906=CARTESIAN_POINT('',(6.,6.25657141382095,-3.29463795232411));
#31907=CARTESIAN_POINT('',(6.,3.05700229224093,-2.25503492526414));
#31908=CARTESIAN_POINT('',(6.,6.99821220032083,-1.01210231321574));
#31909=CARTESIAN_POINT('',(6.,6.81280200369586,-1.58273622299284));
#31910=CARTESIAN_POINT('',(6.,7.60688837074973,-1.20987318961571));
#31911=CARTESIAN_POINT('',(6.,4.27417133688838,-0.127007783343246));
#31912=CARTESIAN_POINT('',(6.,7.92583592135001,-0.228253563910837));
#31913=CARTESIAN_POINT('',(6.,6.47213595499958,-4.70228201833979));
#31914=CARTESIAN_POINT('',(6.,7.92583592135001,0.228253563910837));
#31915=CARTESIAN_POINT('',(6.,7.92583592135001,6.93889390390723E-17));
#31916=CARTESIAN_POINT('',(6.,7.60688837074973,1.20987318961571));
#31917=CARTESIAN_POINT('',(6.,8.,0.));
#31918=CARTESIAN_POINT('',(6.,6.99821220032083,1.01210231321574));
#31919=CARTESIAN_POINT('',(6.,3.7986430787408,-0.0275007138442279));
#31920=CARTESIAN_POINT('',(6.,6.44198161044592,2.72400404254702));
#31921=CARTESIAN_POINT('Origin',(5.88,6.55610839240134,2.76108608187201));
#31922=CARTESIAN_POINT('',(5.76,7.22646576423166,1.08626639186573));
#31923=CARTESIAN_POINT('',(5.13,7.82563136949761,1.28094709832195));
#31924=CARTESIAN_POINT('',(5.76,6.48482497773179,3.3688020309741));
#31925=CARTESIAN_POINT('',(5.76,6.67023517435676,2.79816812119701));
#31926=CARTESIAN_POINT('',(4.88,7.32175471207153,3.64073698602405));
#31927=CARTESIAN_POINT('Origin',(3.,6.48482497773179,3.3688020309741));
#31928=CARTESIAN_POINT('',(3.,7.22646576423166,1.08626639186573));
#31929=CARTESIAN_POINT('',(3.,7.22646576423166,1.08626639186573));
#31930=CARTESIAN_POINT('',(3.,6.48482497773179,3.3688020309741));
#31931=CARTESIAN_POINT('',(3.,7.22646576423166,1.08626639186573));
#31932=CARTESIAN_POINT('',(3.,6.48482497773179,3.3688020309741));
#31933=CARTESIAN_POINT('Origin',(5.88,3.68107742718252,6.08734938865102));
#31934=CARTESIAN_POINT('',(5.76,5.20784224733253,5.12641797384956));
#31935=CARTESIAN_POINT('',(5.13,5.57814695627679,5.63609868030578));
#31936=CARTESIAN_POINT('',(5.76,3.26620146083265,6.53710257935149));
#31937=CARTESIAN_POINT('',(5.76,3.75161165745762,6.18443142797601));
#31938=CARTESIAN_POINT('',(4.88,3.78345248285003,7.24903753440145));
#31939=CARTESIAN_POINT('Origin',(3.,3.26620146083265,6.53710257935149));
#31940=CARTESIAN_POINT('',(3.,5.20784224733253,5.12641797384956));
#31941=CARTESIAN_POINT('',(3.,5.20784224733253,5.12641797384956));
#31942=CARTESIAN_POINT('',(3.,3.26620146083265,6.53710257935149));
#31943=CARTESIAN_POINT('',(3.,5.20784224733253,5.12641797384956));
#31944=CARTESIAN_POINT('',(3.,3.26620146083265,6.53710257935149));
#31945=CARTESIAN_POINT('Origin',(5.88,-0.6,7.08845213036123));
#31946=CARTESIAN_POINT('',(5.76,1.2,7.20845213036123));
#31947=CARTESIAN_POINT('',(5.13,1.2,7.83845213036123));
#31948=CARTESIAN_POINT('',(5.76,-1.2,7.20845213036123));
#31949=CARTESIAN_POINT('',(5.76,-0.6,7.20845213036123));
#31950=CARTESIAN_POINT('',(4.88,-1.2,8.08845213036123));
#31951=CARTESIAN_POINT('Origin',(3.,-1.2,7.20845213036123));
#31952=CARTESIAN_POINT('',(3.,1.2,7.20845213036123));
#31953=CARTESIAN_POINT('',(3.,1.2,7.20845213036123));
#31954=CARTESIAN_POINT('',(3.,-1.2,7.20845213036123));
#31955=CARTESIAN_POINT('',(3.,1.2,7.20845213036123));
#31956=CARTESIAN_POINT('',(3.,-1.2,7.20845213036123));
#31957=CARTESIAN_POINT('Origin',(0.,6.26797976099509,4.55395386103981));
#31958=CARTESIAN_POINT('',(0.24,6.54630003364957,4.47402845442895));
#31959=CARTESIAN_POINT('',(0.24,6.27797187634959,4.84335047888998));
#31960=CARTESIAN_POINT('',(0.24,6.54630003364957,4.47402845442895));
#31961=CARTESIAN_POINT('',(0.,6.26797976099509,4.55395386103981));
#31962=CARTESIAN_POINT('',(0.24,6.27797187634959,4.84335047888998));
#31963=CARTESIAN_POINT('Origin',(0.12,7.50390720679448,1.13848846525995));
#31964=CARTESIAN_POINT('',(0.169465769724903,7.92583592135001,-2.15105711021124E-15));
#31965=CARTESIAN_POINT('',(-0.25546881451245,7.47903325825204,-7.21644966006352E-15));
#31966=CARTESIAN_POINT('',(0.24,7.92583592135001,0.228253563910837));
#31967=CARTESIAN_POINT('',(0.24,7.61803398874989,1.17557050458495));
#31968=CARTESIAN_POINT('',(0.320496691051312,7.92583592135001,0.488746328116681));
#31969=CARTESIAN_POINT('Origin',(0.,2.39415522790368,7.36845213036123));
#31970=CARTESIAN_POINT('',(0.24,2.66630003364957,7.46738366981103));
#31971=CARTESIAN_POINT('',(0.24,2.23213595499958,7.60845213036123));
#31972=CARTESIAN_POINT('',(0.24,2.66630003364957,7.46738366981103));
#31973=CARTESIAN_POINT('',(0.,2.39415522790368,7.36845213036123));
#31974=CARTESIAN_POINT('',(0.24,2.23213595499958,7.60845213036123));
#31975=CARTESIAN_POINT('Origin',(0.12,5.40160172472448,5.33174250702015));
#31976=CARTESIAN_POINT('',(0.24,5.47213595499958,5.42882454634515));
#31977=CARTESIAN_POINT('Origin',(0.,-2.39415522790368,7.36845213036123));
#31978=CARTESIAN_POINT('',(0.24,-2.23213595499958,7.60845213036123));
#31979=CARTESIAN_POINT('',(0.24,-2.66630003364957,7.46738366981104));
#31980=CARTESIAN_POINT('',(0.24,-2.23213595499958,7.60845213036123));
#31981=CARTESIAN_POINT('',(0.,-2.39415522790368,7.36845213036123));
#31982=CARTESIAN_POINT('',(0.24,-2.66630003364957,7.46738366981104));
#31983=CARTESIAN_POINT('Origin',(0.12,1.23606797749979,7.48845213036123));
#31984=CARTESIAN_POINT('',(0.24,1.23606797749979,7.60845213036123));
#31985=CARTESIAN_POINT('Origin',(0.12,-3.40160172472448,6.78482756303088));
#31986=CARTESIAN_POINT('',(0.169465769724903,-6.41213595499958,4.65868946665946));
#31987=CARTESIAN_POINT('',(0.24,-6.27797187634959,4.84335047888998));
#31988=CARTESIAN_POINT('',(0.652102425162462,-5.49410648268598,5.92224863481158));
#31989=CARTESIAN_POINT('',(0.24,-3.47213595499958,6.88190960235587));
#31990=CARTESIAN_POINT('',(-0.255468814512445,-6.05066500742134,4.39606545060548));
#31991=CARTESIAN_POINT('Origin',(0.,-2.44921799432457,7.53791790008613));
#31992=CARTESIAN_POINT('',(0.,-2.23213595499958,7.60845213036123));
#31993=CARTESIAN_POINT('',(0.,-2.66630003364957,7.46738366981104));
#31994=CARTESIAN_POINT('Origin',(0.,2.44921799432457,7.53791790008613));
#31995=CARTESIAN_POINT('',(0.,2.66630003364957,7.46738366981103));
#31996=CARTESIAN_POINT('',(0.,2.23213595499958,7.60845213036123));
#31997=CARTESIAN_POINT('Origin',(0.,6.41213595499958,4.65868946665946));
#31998=CARTESIAN_POINT('',(0.,6.54630003364957,4.47402845442895));
#31999=CARTESIAN_POINT('',(0.,6.27797187634959,4.84335047888998));
#32000=CARTESIAN_POINT('Origin',(0.,6.47213595499958,4.70228201833979));
#32001=CARTESIAN_POINT('',(3.,3.50131556174964,6.86070937710148));
#32002=CARTESIAN_POINT('',(1.5,3.50131556174964,6.86070937710148));
#32003=CARTESIAN_POINT('',(3.,5.44295634824952,5.45002477159954));
#32004=CARTESIAN_POINT('',(3.,5.47213595499958,5.42882454634515));
#32005=CARTESIAN_POINT('',(1.5,5.44295634824952,5.45002477159954));
#32006=CARTESIAN_POINT('Origin',(0.,2.47213595499958,7.60845213036123));
#32007=CARTESIAN_POINT('',(3.,-1.2,7.60845213036123));
#32008=CARTESIAN_POINT('',(1.5,-1.2,7.60845213036123));
#32009=CARTESIAN_POINT('',(3.,1.2,7.60845213036123));
#32010=CARTESIAN_POINT('',(3.,1.23606797749979,7.60845213036123));
#32011=CARTESIAN_POINT('',(1.5,1.2,7.60845213036123));
#32012=CARTESIAN_POINT('Origin',(0.,-2.47213595499958,7.60845213036123));
#32013=CARTESIAN_POINT('',(0.,-6.27797187634959,4.84335047888998));
#32014=CARTESIAN_POINT('',(3.,-5.44295634824952,5.45002477159954));
#32015=CARTESIAN_POINT('',(1.5,-5.44295634824952,5.45002477159954));
#32016=CARTESIAN_POINT('',(3.,-3.50131556174964,6.86070937710148));
#32017=CARTESIAN_POINT('',(3.,-3.47213595499958,6.88190960235587));
#32018=CARTESIAN_POINT('',(1.5,-3.50131556174964,6.86070937710148));
#32019=CARTESIAN_POINT('Origin',(0.,-6.41213595499958,4.65868946665947));
#32020=CARTESIAN_POINT('',(0.24,-6.54630003364956,4.47402845442895));
#32021=CARTESIAN_POINT('',(0.24,-6.54630003364956,4.47402845442895));
#32022=CARTESIAN_POINT('',(0.,-6.54630003364956,4.47402845442895));
#32023=CARTESIAN_POINT('Origin',(0.12,-6.73997518429427,3.48962947442985));
#32024=CARTESIAN_POINT('',(0.24,-7.92583592135001,0.228253563910837));
#32025=CARTESIAN_POINT('',(0.,-7.74764906618282,1.66533453693773E-15));
#32026=CARTESIAN_POINT('',(0.24,-6.85410196624968,3.52671151375484));
#32027=CARTESIAN_POINT('Origin',(5.88,-4.65189782043246,5.38200708590005));
#32028=CARTESIAN_POINT('',(5.76,-3.26620146083265,6.5371025793515));
#32029=CARTESIAN_POINT('',(5.13,-3.63650616977691,7.04678328580771));
#32030=CARTESIAN_POINT('',(5.76,-5.20784224733253,5.12641797384956));
#32031=CARTESIAN_POINT('',(5.76,-4.72243205070756,5.47908912522504));
#32032=CARTESIAN_POINT('',(4.88,-5.7250932693499,5.83835292889952));
#32033=CARTESIAN_POINT('Origin',(3.,-5.20784224733253,5.12641797384956));
#32034=CARTESIAN_POINT('',(3.,-3.26620146083265,6.5371025793515));
#32035=CARTESIAN_POINT('',(3.,-3.26620146083265,6.5371025793515));
#32036=CARTESIAN_POINT('',(3.,-5.20784224733253,5.12641797384956));
#32037=CARTESIAN_POINT('',(3.,-3.26620146083265,6.5371025793515));
#32038=CARTESIAN_POINT('',(3.,-5.20784224733253,5.12641797384956));
#32039=CARTESIAN_POINT('Origin',(5.88,-6.92692878565128,1.61981826231783));
#32040=CARTESIAN_POINT('',(5.76,-6.48482497773179,3.3688020309741));
#32041=CARTESIAN_POINT('',(5.13,-7.08399058299774,3.56348273743032));
#32042=CARTESIAN_POINT('',(5.76,-7.22646576423166,1.08626639186573));
#32043=CARTESIAN_POINT('',(5.76,-7.0410555676067,1.65690030164282));
#32044=CARTESIAN_POINT('',(4.88,-8.0633954985714,1.35820134691568));
#32045=CARTESIAN_POINT('Origin',(3.,-7.22646576423166,1.08626639186573));
#32046=CARTESIAN_POINT('',(3.,-6.48482497773179,3.3688020309741));
#32047=CARTESIAN_POINT('',(3.,-6.48482497773179,3.3688020309741));
#32048=CARTESIAN_POINT('',(3.,-7.22646576423166,1.08626639186573));
#32049=CARTESIAN_POINT('',(3.,-6.48482497773179,3.3688020309741));
#32050=CARTESIAN_POINT('',(3.,-7.22646576423166,1.08626639186573));
#32051=CARTESIAN_POINT('Origin',(5.88,-6.55610839240134,-2.76108608187201));
#32052=CARTESIAN_POINT('',(5.76,-7.22646576423166,-1.08626639186573));
#32053=CARTESIAN_POINT('',(5.13,-7.82563136949761,-1.28094709832194));
#32054=CARTESIAN_POINT('',(5.76,-6.48482497773179,-3.3688020309741));
#32055=CARTESIAN_POINT('',(5.76,-6.67023517435676,-2.79816812119701));
#32056=CARTESIAN_POINT('',(4.88,-7.32175471207152,-3.64073698602405));
#32057=CARTESIAN_POINT('Origin',(3.,-6.48482497773179,-3.3688020309741));
#32058=CARTESIAN_POINT('',(3.,-7.22646576423166,-1.08626639186573));
#32059=CARTESIAN_POINT('',(3.,-7.22646576423166,-1.08626639186573));
#32060=CARTESIAN_POINT('',(3.,-6.48482497773179,-3.3688020309741));
#32061=CARTESIAN_POINT('',(3.,-7.22646576423166,-1.08626639186573));
#32062=CARTESIAN_POINT('',(3.,-6.48482497773179,-3.3688020309741));
#32063=CARTESIAN_POINT('Origin',(5.88,-3.68107742718253,-6.08734938865102));
#32064=CARTESIAN_POINT('',(5.76,-5.20784224733253,-5.12641797384956));
#32065=CARTESIAN_POINT('',(5.13,-5.57814695627679,-5.63609868030578));
#32066=CARTESIAN_POINT('',(5.76,-3.26620146083265,-6.53710257935149));
#32067=CARTESIAN_POINT('',(5.76,-3.75161165745762,-6.18443142797601));
#32068=CARTESIAN_POINT('',(4.88,-3.78345248285003,-7.24903753440145));
#32069=CARTESIAN_POINT('Origin',(3.,-3.26620146083265,-6.53710257935149));
#32070=CARTESIAN_POINT('',(3.,-5.20784224733253,-5.12641797384956));
#32071=CARTESIAN_POINT('',(3.,-5.20784224733253,-5.12641797384956));
#32072=CARTESIAN_POINT('',(3.,-3.26620146083265,-6.53710257935149));
#32073=CARTESIAN_POINT('',(3.,-5.20784224733253,-5.12641797384956));
#32074=CARTESIAN_POINT('',(3.,-3.26620146083265,-6.53710257935149));
#32075=CARTESIAN_POINT('Origin',(5.88,0.6,-7.08845213036123));
#32076=CARTESIAN_POINT('',(5.76,-1.2,-7.20845213036123));
#32077=CARTESIAN_POINT('',(5.13,-1.2,-7.83845213036123));
#32078=CARTESIAN_POINT('',(5.76,1.2,-7.20845213036123));
#32079=CARTESIAN_POINT('',(5.76,0.6,-7.20845213036123));
#32080=CARTESIAN_POINT('',(4.88,1.2,-8.08845213036123));
#32081=CARTESIAN_POINT('Origin',(3.,1.2,-7.20845213036123));
#32082=CARTESIAN_POINT('',(3.,-1.2,-7.20845213036123));
#32083=CARTESIAN_POINT('',(3.,-1.2,-7.20845213036123));
#32084=CARTESIAN_POINT('',(3.,1.2,-7.20845213036123));
#32085=CARTESIAN_POINT('',(3.,-1.2,-7.20845213036123));
#32086=CARTESIAN_POINT('',(3.,1.2,-7.20845213036123));
#32087=CARTESIAN_POINT('Origin',(5.88,4.65189782043246,-5.38200708590005));
#32088=CARTESIAN_POINT('',(5.76,3.26620146083265,-6.5371025793515));
#32089=CARTESIAN_POINT('',(5.13,3.63650616977691,-7.04678328580771));
#32090=CARTESIAN_POINT('',(5.76,5.20784224733253,-5.12641797384956));
#32091=CARTESIAN_POINT('',(5.76,4.72243205070756,-5.47908912522504));
#32092=CARTESIAN_POINT('',(4.88,5.7250932693499,-5.83835292889952));
#32093=CARTESIAN_POINT('Origin',(3.,5.20784224733253,-5.12641797384956));
#32094=CARTESIAN_POINT('',(3.,3.26620146083265,-6.5371025793515));
#32095=CARTESIAN_POINT('',(3.,3.26620146083265,-6.5371025793515));
#32096=CARTESIAN_POINT('',(3.,5.20784224733253,-5.12641797384956));
#32097=CARTESIAN_POINT('',(3.,3.26620146083265,-6.5371025793515));
#32098=CARTESIAN_POINT('',(3.,5.20784224733253,-5.12641797384956));
#32099=CARTESIAN_POINT('Origin',(0.,-7.74764906618282,1.66533453693773E-15));
#32100=CARTESIAN_POINT('',(0.24,-7.92583592135001,-0.228253563910836));
#32101=CARTESIAN_POINT('',(0.24,-7.92583592135001,0.228253563910838));
#32102=CARTESIAN_POINT('',(0.24,-7.92583592135001,-0.228253563910836));
#32103=CARTESIAN_POINT('Origin',(0.,-6.26797976099509,-4.55395386103981));
#32104=CARTESIAN_POINT('',(0.24,-6.54630003364957,-4.47402845442895));
#32105=CARTESIAN_POINT('',(0.24,-6.27797187634959,-4.84335047888998));
#32106=CARTESIAN_POINT('',(0.24,-6.54630003364957,-4.47402845442895));
#32107=CARTESIAN_POINT('',(0.,-6.26797976099509,-4.55395386103981));
#32108=CARTESIAN_POINT('',(0.24,-6.27797187634959,-4.84335047888998));
#32109=CARTESIAN_POINT('Origin',(0.12,-7.50390720679448,-1.13848846525995));
#32110=CARTESIAN_POINT('',(0.24,-7.61803398874989,-1.17557050458495));
#32111=CARTESIAN_POINT('Origin',(0.,-2.39415522790368,-7.36845213036123));
#32112=CARTESIAN_POINT('',(0.24,-2.66630003364957,-7.46738366981104));
#32113=CARTESIAN_POINT('',(0.24,-2.23213595499958,-7.60845213036123));
#32114=CARTESIAN_POINT('',(0.24,-2.66630003364957,-7.46738366981103));
#32115=CARTESIAN_POINT('',(0.,-2.39415522790368,-7.36845213036123));
#32116=CARTESIAN_POINT('',(0.24,-2.23213595499958,-7.60845213036123));
#32117=CARTESIAN_POINT('Origin',(0.12,-5.40160172472448,-5.33174250702015));
#32118=CARTESIAN_POINT('',(0.24,-5.47213595499958,-5.42882454634514));
#32119=CARTESIAN_POINT('Origin',(0.,2.39415522790368,-7.36845213036123));
#32120=CARTESIAN_POINT('',(0.24,2.23213595499958,-7.60845213036123));
#32121=CARTESIAN_POINT('',(0.24,2.66630003364957,-7.46738366981103));
#32122=CARTESIAN_POINT('',(0.24,2.23213595499958,-7.60845213036123));
#32123=CARTESIAN_POINT('',(0.,2.39415522790368,-7.36845213036123));
#32124=CARTESIAN_POINT('',(0.24,2.66630003364957,-7.46738366981103));
#32125=CARTESIAN_POINT('Origin',(0.12,-1.23606797749979,-7.48845213036123));
#32126=CARTESIAN_POINT('',(0.24,-1.23606797749979,-7.60845213036123));
#32127=CARTESIAN_POINT('Origin',(0.24,6.54630003364957,-4.47402845442895));
#32128=CARTESIAN_POINT('',(0.24,6.27797187634959,-4.84335047888998));
#32129=CARTESIAN_POINT('',(0.,6.26797976099509,-4.55395386103981));
#32130=CARTESIAN_POINT('',(0.24,6.54630003364957,-4.47402845442895));
#32131=CARTESIAN_POINT('',(0.24,6.54630003364957,-4.47402845442895));
#32132=CARTESIAN_POINT('',(0.24,6.27797187634959,-4.84335047888998));
#32133=CARTESIAN_POINT('Origin',(0.12,6.73997518429427,-3.48962947442985));
#32134=CARTESIAN_POINT('',(0.24,7.92583592135001,-0.228253563910837));
#32135=CARTESIAN_POINT('',(0.0989315394498051,7.92583592135001,0.228253563910837));
#32136=CARTESIAN_POINT('',(0.24,6.85410196624968,-3.52671151375484));
#32137=CARTESIAN_POINT('Origin',(0.,6.41213595499958,-4.65868946665946));
#32138=CARTESIAN_POINT('',(0.,6.27797187634959,-4.84335047888998));
#32139=CARTESIAN_POINT('',(0.,6.54630003364957,-4.47402845442895));
#32140=CARTESIAN_POINT('Origin',(0.12,3.40160172472448,-6.78482756303088));
#32141=CARTESIAN_POINT('',(0.24,3.47213595499958,-6.88190960235587));
#32142=CARTESIAN_POINT('Origin',(0.,7.92583592135001,1.38777878078145E-16));
#32143=CARTESIAN_POINT('',(0.,7.92583592135001,0.228253563910837));
#32144=CARTESIAN_POINT('',(0.,7.92583592135001,-0.228253563910837));
#32145=CARTESIAN_POINT('Origin',(0.,2.44921799432457,-7.53791790008613));
#32146=CARTESIAN_POINT('',(0.,2.23213595499958,-7.60845213036123));
#32147=CARTESIAN_POINT('',(0.,2.66630003364957,-7.46738366981103));
#32148=CARTESIAN_POINT('Origin',(0.,-2.44921799432457,-7.53791790008613));
#32149=CARTESIAN_POINT('',(0.,-2.66630003364957,-7.46738366981103));
#32150=CARTESIAN_POINT('',(0.,-2.23213595499958,-7.60845213036123));
#32151=CARTESIAN_POINT('Origin',(0.,-6.41213595499958,-4.65868946665946));
#32152=CARTESIAN_POINT('',(0.,-6.54630003364957,-4.47402845442895));
#32153=CARTESIAN_POINT('',(0.,-6.27797187634959,-4.84335047888998));
#32154=CARTESIAN_POINT('Origin',(0.,-7.92583592135001,9.36750677027476E-16));
#32155=CARTESIAN_POINT('',(0.,-7.92583592135001,0.228253563910838));
#32156=CARTESIAN_POINT('',(0.,-7.92583592135001,-0.228253563910836));
#32157=CARTESIAN_POINT('Origin',(0.,-6.47213595499958,4.70228201833979));
#32158=CARTESIAN_POINT('',(3.,-7.60688837074973,1.20987318961571));
#32159=CARTESIAN_POINT('',(1.5,-7.60688837074973,1.20987318961571));
#32160=CARTESIAN_POINT('',(3.,-6.86524758424985,3.49240882872408));
#32161=CARTESIAN_POINT('',(3.,-6.85410196624968,3.52671151375484));
#32162=CARTESIAN_POINT('',(1.5,-6.86524758424985,3.49240882872408));
#32163=CARTESIAN_POINT('Origin',(0.,-8.,9.79717439317883E-16));
#32164=CARTESIAN_POINT('',(3.,-6.86524758424985,-3.49240882872408));
#32165=CARTESIAN_POINT('',(1.5,-6.86524758424985,-3.49240882872408));
#32166=CARTESIAN_POINT('',(3.,-7.60688837074973,-1.20987318961571));
#32167=CARTESIAN_POINT('',(3.,-7.61803398874989,-1.17557050458495));
#32168=CARTESIAN_POINT('',(1.5,-7.60688837074973,-1.20987318961571));
#32169=CARTESIAN_POINT('Origin',(0.,-6.47213595499958,-4.70228201833978));
#32170=CARTESIAN_POINT('',(3.,-3.50131556174964,-6.86070937710147));
#32171=CARTESIAN_POINT('',(1.5,-3.50131556174964,-6.86070937710147));
#32172=CARTESIAN_POINT('',(3.,-5.44295634824952,-5.45002477159954));
#32173=CARTESIAN_POINT('',(3.,-5.47213595499958,-5.42882454634515));
#32174=CARTESIAN_POINT('',(1.5,-5.44295634824952,-5.45002477159954));
#32175=CARTESIAN_POINT('Origin',(0.,-2.47213595499958,-7.60845213036123));
#32176=CARTESIAN_POINT('',(3.,1.2,-7.60845213036123));
#32177=CARTESIAN_POINT('',(1.5,1.2,-7.60845213036123));
#32178=CARTESIAN_POINT('',(3.,-1.2,-7.60845213036123));
#32179=CARTESIAN_POINT('',(3.,-1.23606797749979,-7.60845213036123));
#32180=CARTESIAN_POINT('',(1.5,-1.2,-7.60845213036123));
#32181=CARTESIAN_POINT('Origin',(0.,2.47213595499958,-7.60845213036123));
#32182=CARTESIAN_POINT('',(3.,5.44295634824952,-5.45002477159954));
#32183=CARTESIAN_POINT('',(1.5,5.44295634824952,-5.45002477159954));
#32184=CARTESIAN_POINT('',(3.,3.50131556174964,-6.86070937710148));
#32185=CARTESIAN_POINT('',(3.,3.47213595499958,-6.88190960235587));
#32186=CARTESIAN_POINT('',(1.5,3.50131556174964,-6.86070937710148));
#32187=CARTESIAN_POINT('Origin',(5.88,6.92692878565128,-1.61981826231783));
#32188=CARTESIAN_POINT('',(5.76,6.48482497773179,-3.3688020309741));
#32189=CARTESIAN_POINT('',(5.13,7.08399058299774,-3.56348273743032));
#32190=CARTESIAN_POINT('',(5.76,7.22646576423166,-1.08626639186573));
#32191=CARTESIAN_POINT('',(5.76,7.0410555676067,-1.65690030164282));
#32192=CARTESIAN_POINT('',(4.88,8.0633954985714,-1.35820134691568));
#32193=CARTESIAN_POINT('Origin',(3.,7.22646576423166,-1.08626639186573));
#32194=CARTESIAN_POINT('',(3.,6.48482497773179,-3.3688020309741));
#32195=CARTESIAN_POINT('',(3.,6.48482497773179,-3.3688020309741));
#32196=CARTESIAN_POINT('',(3.,7.22646576423166,-1.08626639186573));
#32197=CARTESIAN_POINT('',(3.,6.48482497773179,-3.3688020309741));
#32198=CARTESIAN_POINT('',(3.,7.22646576423166,-1.08626639186573));
#32199=CARTESIAN_POINT('Origin',(3.,7.3311736291293,-2.38204270860739));
#32200=CARTESIAN_POINT('',(3.,7.60688837074973,-1.20987318961571));
#32201=CARTESIAN_POINT('',(3.,6.86524758424985,-3.49240882872408));
#32202=CARTESIAN_POINT('',(3.,6.85410196624968,-3.52671151375484));
#32203=CARTESIAN_POINT('',(3.,7.22646576423166,-1.08626639186573));
#32204=CARTESIAN_POINT('',(3.,7.43588149402694,-3.67781902534905));
#32205=CARTESIAN_POINT('Origin',(3.,6.48482497773179,-3.3688020309741));
#32206=CARTESIAN_POINT('',(1.5,6.86524758424985,-3.49240882872408));
#32207=CARTESIAN_POINT('Origin',(3.,8.17752228052682,-1.39528338624068));
#32208=CARTESIAN_POINT('',(1.5,7.60688837074973,-1.20987318961571));
#32209=CARTESIAN_POINT('Origin',(0.,6.47213595499958,-4.70228201833979));
#32210=CARTESIAN_POINT('Origin',(3.,4.53091448022882,-6.236268773788));
#32211=CARTESIAN_POINT('',(3.,5.20784224733253,-5.12641797384956));
#32212=CARTESIAN_POINT('',(3.,3.85398671312512,-7.34611957372644));
#32213=CARTESIAN_POINT('Origin',(3.,3.26620146083265,-6.5371025793515));
#32214=CARTESIAN_POINT('Origin',(3.,5.795627499625,-5.93543496822451));
#32215=CARTESIAN_POINT('Origin',(3.,-1.38777878078145E-15,-7.70845213036123));
#32216=CARTESIAN_POINT('',(3.,1.2,-7.20845213036123));
#32217=CARTESIAN_POINT('',(3.,-1.2,-8.20845213036123));
#32218=CARTESIAN_POINT('Origin',(3.,-1.2,-7.20845213036123));
#32219=CARTESIAN_POINT('Origin',(3.,1.2,-8.20845213036123));
#32220=CARTESIAN_POINT('Origin',(3.,-4.53091448022883,-6.236268773788));
#32221=CARTESIAN_POINT('',(3.,-3.26620146083265,-6.53710257935149));
#32222=CARTESIAN_POINT('',(3.,-5.795627499625,-5.93543496822451));
#32223=CARTESIAN_POINT('Origin',(3.,-5.20784224733253,-5.12641797384956));
#32224=CARTESIAN_POINT('Origin',(3.,-3.85398671312513,-7.34611957372644));
#32225=CARTESIAN_POINT('Origin',(3.,-7.3311736291293,-2.38204270860739));
#32226=CARTESIAN_POINT('',(3.,-6.48482497773179,-3.3688020309741));
#32227=CARTESIAN_POINT('',(3.,-8.17752228052682,-1.39528338624068));
#32228=CARTESIAN_POINT('Origin',(3.,-7.22646576423166,-1.08626639186573));
#32229=CARTESIAN_POINT('Origin',(3.,-7.43588149402694,-3.67781902534904));
#32230=CARTESIAN_POINT('Origin',(3.,-7.3311736291293,2.38204270860739));
#32231=CARTESIAN_POINT('',(3.,-7.22646576423166,1.08626639186573));
#32232=CARTESIAN_POINT('',(3.,-7.43588149402694,3.67781902534905));
#32233=CARTESIAN_POINT('Origin',(3.,-6.48482497773179,3.3688020309741));
#32234=CARTESIAN_POINT('Origin',(3.,-8.17752228052682,1.39528338624068));
#32235=CARTESIAN_POINT('Origin',(3.,-4.53091448022883,6.236268773788));
#32236=CARTESIAN_POINT('',(3.,-5.20784224733253,5.12641797384956));
#32237=CARTESIAN_POINT('',(3.,-3.85398671312513,7.34611957372644));
#32238=CARTESIAN_POINT('Origin',(3.,-3.26620146083265,6.5371025793515));
#32239=CARTESIAN_POINT('Origin',(3.,-5.795627499625,5.93543496822451));
#32240=CARTESIAN_POINT('Origin',(3.,5.55111512312578E-16,7.70845213036123));
#32241=CARTESIAN_POINT('',(3.,-1.2,7.20845213036123));
#32242=CARTESIAN_POINT('',(3.,1.2,8.20845213036123));
#32243=CARTESIAN_POINT('Origin',(3.,1.2,7.20845213036123));
#32244=CARTESIAN_POINT('Origin',(3.,-1.2,8.20845213036123));
#32245=CARTESIAN_POINT('Origin',(3.,4.53091448022883,6.236268773788));
#32246=CARTESIAN_POINT('',(3.,3.26620146083265,6.53710257935149));
#32247=CARTESIAN_POINT('',(3.,5.795627499625,5.93543496822451));
#32248=CARTESIAN_POINT('Origin',(3.,5.20784224733253,5.12641797384956));
#32249=CARTESIAN_POINT('Origin',(3.,3.85398671312513,7.34611957372644));
#32250=CARTESIAN_POINT('Origin',(3.,7.22646576423166,1.08626639186573));
#32251=CARTESIAN_POINT('',(3.,7.60688837074973,1.20987318961571));
#32252=CARTESIAN_POINT('',(1.5,7.60688837074973,1.20987318961571));
#32253=CARTESIAN_POINT('',(3.,8.17752228052682,1.39528338624068));
#32254=CARTESIAN_POINT('Origin',(3.,7.43588149402694,3.67781902534904));
#32255=CARTESIAN_POINT('',(3.,6.86524758424985,3.49240882872408));
#32256=CARTESIAN_POINT('',(1.5,6.86524758424985,3.49240882872408));
#32257=CARTESIAN_POINT('',(3.,6.48482497773179,3.3688020309741));
#32258=CARTESIAN_POINT('Origin',(3.,7.3311736291293,2.38204270860739));
#32259=CARTESIAN_POINT('',(3.,7.61803398874989,1.17557050458495));
#32260=CARTESIAN_POINT('Origin',(0.,8.,0.));
#32292=UNCERTAINTY_MEASURE_WITH_UNIT(LENGTH_MEASURE(0.01),#32310,
'DISTANCE_ACCURACY_VALUE',
'Maximum model space distance between geometric entities at asserted c
onnectivities');
#32293=UNCERTAINTY_MEASURE_WITH_UNIT(LENGTH_MEASURE(0.01),#32310,
'DISTANCE_ACCURACY_VALUE',
'Maximum model space distance between geometric entities at asserted c
onnectivities');
#32308=(
GEOMETRIC_REPRESENTATION_CONTEXT(3)
GLOBAL_UNCERTAINTY_ASSIGNED_CONTEXT((#32292))
GLOBAL_UNIT_ASSIGNED_CONTEXT((#32310,#32312,#32313))
REPRESENTATION_CONTEXT('','3D')
);
#32309=(
GEOMETRIC_REPRESENTATION_CONTEXT(3)
GLOBAL_UNCERTAINTY_ASSIGNED_CONTEXT((#32293))
GLOBAL_UNIT_ASSIGNED_CONTEXT((#32310,#32312,#32313))
REPRESENTATION_CONTEXT('','3D')
);
#32310=(
LENGTH_UNIT()
NAMED_UNIT(*)
SI_UNIT(.MILLI.,.METRE.)
);
#32312=(
NAMED_UNIT(*)
PLANE_ANGLE_UNIT()
SI_UNIT($,.RADIAN.)
);
#32313=(
NAMED_UNIT(*)
SI_UNIT($,.STERADIAN.)
SOLID_ANGLE_UNIT()
);
#32328=SHAPE_DEFINITION_REPRESENTATION(#32343,#32375);
#32343=PRODUCT_DEFINITION_SHAPE('',$,#32391);
#32375=SHAPE_REPRESENTATION('',(#14889),#32308);
#32376=PRODUCT_DEFINITION_CONTEXT('part definition',#32423,'design');
#32391=PRODUCT_DEFINITION('2026-10-25-00-35-19-921',
'10_Combination_Dial_Wheel',#32406,#32376);
#32406=PRODUCT_DEFINITION_FORMATION('',$,#32439);
#32423=APPLICATION_CONTEXT(
'Core Data for Automotive Mechanical Design Process');
#32424=PRODUCT_CONTEXT('part definition',#32423,'mechanical');
#32439=PRODUCT('2026-10-25-00-35-19-921','10_Combination_Dial_Wheel',$,
(#32424));
#32482=COLOUR_RGB('Light Blue',0.38,0.62,0.78);
#32483=FILL_AREA_STYLE_COLOUR('',#32482);
#32484=FILL_AREA_STYLE('',(#32483));
#32485=SURFACE_STYLE_FILL_AREA(#32484);
#32486=SURFACE_SIDE_STYLE('',(#32485));
#32487=SURFACE_STYLE_USAGE(.BOTH.,#32486);
#32488=PRESENTATION_STYLE_ASSIGNMENT((#32487));
ENDSEC;
END-ISO-10303-21;
